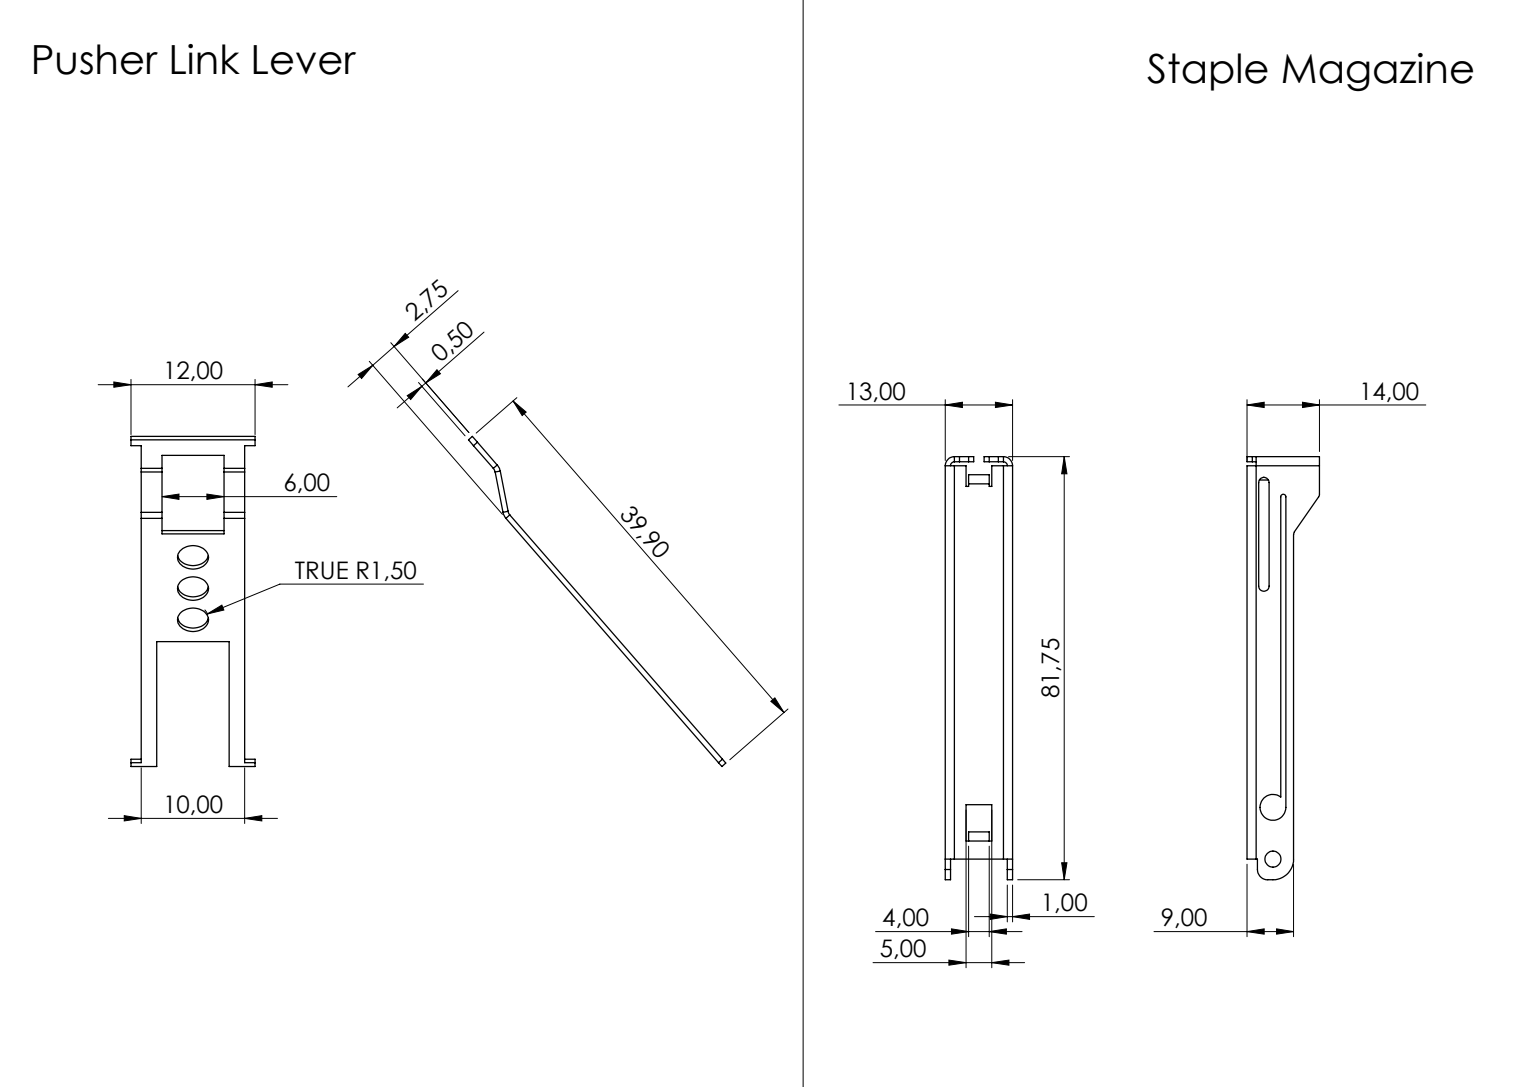
ISO-10303-21;
HEADER;
FILE_DESCRIPTION (('STEP AP214'),
    '1' );
FILE_NAME ('Staple Magazine.step',
    '2026-10-06T10:23:46',
    ( '' ),
    ( '' ),
    'SwSTEP 2.0',
    'SolidWorks 2020',
    '' );
FILE_SCHEMA (( 'AUTOMOTIVE_DESIGN' ));
ENDSEC;

DATA;
#2=ORIENTED_EDGE ( 'NONE', *, *, #5924, .T. ) ;
#11=DIRECTION ( 'NONE',  ( -6.056754644426120895E-31, -1.000000000000000000, -4.914813388431354887E-16 ) ) ;
#25=DIRECTION ( 'NONE',  ( 8.673617379884039170E-17, 2.999999999999999839E-15, 1.000000000000000000 ) ) ;
#29=EDGE_LOOP ( 'NONE', ( #453, #19107 ) ) ;
#33=CARTESIAN_POINT ( 'NONE',  ( 40.81606138205700773, -31.05876147765399864, 75.30501292737010033 ) ) ;
#40=CARTESIAN_POINT ( 'NONE',  ( 42.06606138205700063, 43.19123852234599781, 75.30501292736987295 ) ) ;
#46=( NAMED_UNIT ( * ) SI_UNIT ( $, .STERADIAN. ) SOLID_ANGLE_UNIT ( ) );
#53=ORIENTED_EDGE ( 'NONE', *, *, #21241, .F. ) ;
#64=VERTEX_POINT ( 'NONE', #911 ) ;
#66=EDGE_CURVE ( 'NONE', #3119, #2388, #6890, .T. ) ;
#78=FACE_BOUND ( 'NONE', #23310, .T. ) ;
#90=ORIENTED_EDGE ( 'NONE', *, *, #479, .T. ) ;
#93=AXIS2_PLACEMENT_3D ( 'NONE', #14032, #16324, #20207 ) ;
#94=EDGE_CURVE ( 'NONE', #4444, #1424, #20510, .T. ) ;
#95=DIRECTION ( 'NONE',  ( 1.000000000000000000, 0.000000000000000000, 0.000000000000000000 ) ) ;
#103=DIRECTION ( 'NONE',  ( 2.312964634635740294E-15, 2.999999999999999839E-15, 1.000000000000000000 ) ) ;
#108=VECTOR ( 'NONE', #19668, 1000.000000000000000 ) ;
#116=CARTESIAN_POINT ( 'NONE',  ( 44.81606138205700063, -24.55876147765401285, 70.30501292737008612 ) ) ;
#118=CYLINDRICAL_SURFACE ( 'NONE', #9476, 1.000000000000000888 ) ;
#132=AXIS2_PLACEMENT_3D ( 'NONE', #6490, #16519, #18844 ) ;
#141=EDGE_CURVE ( 'NONE', #14226, #13391, #3231, .T. ) ;
#150=AXIS2_PLACEMENT_3D ( 'NONE', #11257, #7991, #1314 ) ;
#154=VERTEX_POINT ( 'NONE', #12549 ) ;
#157=CARTESIAN_POINT ( 'NONE',  ( 36.31606138205700063, 39.69123852234597649, 69.30501292736988717 ) ) ;
#164=CIRCLE ( 'NONE', #21962, 1.000000000000000888 ) ;
#177=ORIENTED_EDGE ( 'NONE', *, *, #13046, .F. ) ;
#179=DIRECTION ( 'NONE',  ( 1.000000000000000000, -5.204170427930413997E-31, -1.734723475976804876E-16 ) ) ;
#186=ORIENTED_EDGE ( 'NONE', *, *, #12634, .T. ) ;
#197=VECTOR ( 'NONE', #7883, 1000.000000000000000 ) ;
#201=CARTESIAN_POINT ( 'NONE',  ( 44.81606138205700063, 41.44123852234595518, 61.30501292736988006 ) ) ;
#207=CARTESIAN_POINT ( 'NONE',  ( 40.31606138205700773, 37.94123852234599070, 73.55501292736988717 ) ) ;
#210=LINE ( 'NONE', #8213, #17640 ) ;
#216=EDGE_LOOP ( 'NONE', ( #18034, #25103, #6817, #21837 ) ) ;
#221=ORIENTED_EDGE ( 'NONE', *, *, #10919, .F. ) ;
#222=DIRECTION ( 'NONE',  ( 0.000000000000000000, -2.999999999999999839E-15, -1.000000000000000000 ) ) ;
#244=LINE ( 'NONE', #4267, #5670 ) ;
#245=EDGE_CURVE ( 'NONE', #15791, #17958, #9316, .T. ) ;
#254=CYLINDRICAL_SURFACE ( 'NONE', #13248, 1.000000000000000888 ) ;
#268=DIRECTION ( 'NONE',  ( 1.000000000000000000, 3.083952846180988900E-15, -3.854941057726327830E-16 ) ) ;
#270=CIRCLE ( 'NONE', #24538, 2.000000000000001776 ) ;
#278=ORIENTED_EDGE ( 'NONE', *, *, #24831, .T. ) ;
#285=CARTESIAN_POINT ( 'NONE',  ( 44.81606138205700063, -34.55876147765400930, 73.30501292737011454 ) ) ;
#293=CARTESIAN_POINT ( 'NONE',  ( 40.31606138205700773, 39.69123852234597649, 69.30501292736988717 ) ) ;
#294=DIRECTION ( 'NONE',  ( 0.000000000000000000, 2.775557561562888984E-15, 1.000000000000000000 ) ) ;
#297=DIRECTION ( 'NONE',  ( 0.000000000000000000, -2.999999999999999839E-15, -1.000000000000000000 ) ) ;
#302=FACE_OUTER_BOUND ( 'NONE', #11083, .T. ) ;
#304=ADVANCED_FACE ( 'NONE', ( #3366 ), #21151, .F. ) ;
#314=ORIENTED_EDGE ( 'NONE', *, *, #23269, .F. ) ;
#316=CARTESIAN_POINT ( 'NONE',  ( 40.31606138205700773, 38.69123852234599070, 73.55501292736988717 ) ) ;
#317=CARTESIAN_POINT ( 'NONE',  ( 31.81606138205700418, -24.55876147765401285, 70.30501292737008612 ) ) ;
#324=ORIENTED_EDGE ( 'NONE', *, *, #10135, .F. ) ;
#325=ORIENTED_EDGE ( 'NONE', *, *, #16629, .F. ) ;
#328=CARTESIAN_POINT ( 'NONE',  ( 31.81606138205700418, 28.69846577177642288, 66.12638289304319983 ) ) ;
#335=PLANE ( 'NONE',  #18029 ) ;
#342=ORIENTED_EDGE ( 'NONE', *, *, #16102, .F. ) ;
#347=DIRECTION ( 'NONE',  ( -3.717264591378870232E-16, -3.325260651745651169E-15, -1.000000000000000000 ) ) ;
#355=CARTESIAN_POINT ( 'NONE',  ( 33.56606138205700773, 41.44123852234599070, 73.55501292736987295 ) ) ;
#357=FACE_OUTER_BOUND ( 'NONE', #24183, .T. ) ;
#359=VECTOR ( 'NONE', #22680, 1000.000000000000000 ) ;
#363=EDGE_LOOP ( 'NONE', ( #20532, #24029, #12910, #14891, #19447, #20167, #13360, #10230, #14079, #1336, #8917 ) ) ;
#364=ORIENTED_EDGE ( 'NONE', *, *, #2300, .T. ) ;
#375=ADVANCED_FACE ( 'NONE', ( #8387 ), #5942, .F. ) ;
#384=CARTESIAN_POINT ( 'NONE',  ( 40.31606138205700773, 41.44123852234599781, 74.30501292736987295 ) ) ;
#392=CARTESIAN_POINT ( 'NONE',  ( 44.81606138205700063, -38.55876147765400930, 73.30501292737012875 ) ) ;
#409=EDGE_CURVE ( 'NONE', #17565, #5522, #244, .T. ) ;
#412=LINE ( 'NONE', #17964, #14177 ) ;
#428=ADVANCED_FACE ( 'NONE', ( #6197 ), #2308, .T. ) ;
#431=CARTESIAN_POINT ( 'NONE',  ( 36.31606138205700063, -30.30876147765400574, 73.55501292737010033 ) ) ;
#443=LINE ( 'NONE', #18607, #21420 ) ;
#444=LINE ( 'NONE', #22224, #5450 ) ;
#449=CARTESIAN_POINT ( 'NONE',  ( 35.31606138205687273, 42.19123852234595518, 61.80501292736988006 ) ) ;
#453=ORIENTED_EDGE ( 'NONE', *, *, #20893, .T. ) ;
#456=CARTESIAN_POINT ( 'NONE',  ( 36.31606138205700063, 43.19123852234599781, 74.30501292736987295 ) ) ;
#466=CARTESIAN_POINT ( 'NONE',  ( 33.56606138205700773, 43.19123852234599781, 75.30501292736987295 ) ) ;
#472=AXIS2_PLACEMENT_3D ( 'NONE', #1050, #9195, #18717 ) ;
#473=CARTESIAN_POINT ( 'NONE',  ( 31.81606138205700418, -22.55876147765401996, 68.80501292737008612 ) ) ;
#478=FACE_OUTER_BOUND ( 'NONE', #5733, .T. ) ;
#479=EDGE_CURVE ( 'NONE', #15938, #12825, #16471, .T. ) ;
#504=VECTOR ( 'NONE', #8993, 1000.000000000000000 ) ;
#515=CARTESIAN_POINT ( 'NONE',  ( 32.81606138205700773, 35.38401127291550097, 61.48364296169660292 ) ) ;
#518=AXIS2_PLACEMENT_3D ( 'NONE', #8054, #21699, #12437 ) ;
#531=FACE_OUTER_BOUND ( 'NONE', #15557, .T. ) ;
#537=FACE_OUTER_BOUND ( 'NONE', #20506, .T. ) ;
#540=CIRCLE ( 'NONE', #15353, 0.9999999999999940048 ) ;
#541=CARTESIAN_POINT ( 'NONE',  ( 31.81606138205700418, 38.19123852234599070, 72.05501292736988717 ) ) ;
#549=VECTOR ( 'NONE', #9794, 1000.000000000000000 ) ;
#555=AXIS2_PLACEMENT_3D ( 'NONE', #19698, #6310, #13908 ) ;
#570=DIRECTION ( 'NONE',  ( 0.000000000000000000, 1.000000000000000000, -2.999999999999999839E-15 ) ) ;
#595=DIRECTION ( 'NONE',  ( -1.836970198721029688E-16, -2.999999999999999839E-15, -1.000000000000000000 ) ) ;
#596=DIRECTION ( 'NONE',  ( 1.000000000000000000, -5.204170427930415223E-30, -1.734723475976805122E-15 ) ) ;
#620=ORIENTED_EDGE ( 'NONE', *, *, #4318, .T. ) ;
#646=ADVANCED_FACE ( 'NONE', ( #14389 ), #335, .T. ) ;
#652=EDGE_LOOP ( 'NONE', ( #17580, #11877, #24697, #22252 ) ) ;
#663=DIRECTION ( 'NONE',  ( 1.000000000000000000, 0.000000000000000000, 0.000000000000000000 ) ) ;
#665=LINE ( 'NONE', #21852, #15394 ) ;
#667=FACE_OUTER_BOUND ( 'NONE', #25437, .T. ) ;
#673=CARTESIAN_POINT ( 'NONE',  ( 34.56606138205700773, 41.44123852234599781, 74.30501292736987295 ) ) ;
#675=CARTESIAN_POINT ( 'NONE',  ( 36.31606138205700063, 37.44123852234599781, 74.30501292736988717 ) ) ;
#685=UNCERTAINTY_MEASURE_WITH_UNIT (LENGTH_MEASURE( 1.000000000000000082E-05 ), #25478, 'distance_accuracy_value', 'NONE');
#701=ORIENTED_EDGE ( 'NONE', *, *, #6875, .T. ) ;
#707=DIRECTION ( 'NONE',  ( -9.027796614315171564E-31, -1.000000000000000000, -3.938893903907230117E-15 ) ) ;
#712=VECTOR ( 'NONE', #15259, 1000.000000000000000 ) ;
#716=ORIENTED_EDGE ( 'NONE', *, *, #3484, .F. ) ;
#717=EDGE_CURVE ( 'NONE', #11800, #9537, #10630, .T. ) ;
#719=DIRECTION ( 'NONE',  ( 1.000000000000000000, 0.000000000000000000, 0.000000000000000000 ) ) ;
#737=DIRECTION ( 'NONE',  ( 3.469446951953614978E-15, 2.999999999999999839E-15, 1.000000000000000000 ) ) ;
#738=CARTESIAN_POINT ( 'NONE',  ( 44.81606138205700063, 18.19123852234599426, 73.05501292736995822 ) ) ;
#741=CARTESIAN_POINT ( 'NONE',  ( 31.81606138205700418, 38.19123852234599070, 73.05501292736988717 ) ) ;
#744=LINE ( 'NONE', #10175, #2475 ) ;
#745=ORIENTED_EDGE ( 'NONE', *, *, #978, .F. ) ;
#763=FACE_OUTER_BOUND ( 'NONE', #937, .T. ) ;
#767=ADVANCED_FACE ( 'NONE', ( #6412 ), #16191, .F. ) ;
#795=FACE_OUTER_BOUND ( 'NONE', #17917, .T. ) ;
#796=EDGE_CURVE ( 'NONE', #6775, #12825, #1233, .T. ) ;
#811=VECTOR ( 'NONE', #1544, 1000.000000000000000 ) ;
#821=VERTEX_POINT ( 'NONE', #16699 ) ;
#824=DIRECTION ( 'NONE',  ( 0.000000000000000000, -1.000000000000000000, 2.999999999999999839E-15 ) ) ;
#826=CARTESIAN_POINT ( 'NONE',  ( 31.81606138205700418, -34.55876147765401640, 70.30501292737011454 ) ) ;
#837=DIRECTION ( 'NONE',  ( -1.000000000000000000, 1.115179377413661005E-30, 3.717264591378870232E-16 ) ) ;
#842=ORIENTED_EDGE ( 'NONE', *, *, #1376, .F. ) ;
#875=DIRECTION ( 'NONE',  ( 3.491481338843135327E-15, 1.000000000000000000, -3.000000000000000628E-15 ) ) ;
#879=ORIENTED_EDGE ( 'NONE', *, *, #18939, .T. ) ;
#880=CIRCLE ( 'NONE', #9142, 1.000000000000000888 ) ;
#881=EDGE_CURVE ( 'NONE', #23679, #25358, #20565, .T. ) ;
#911=CARTESIAN_POINT ( 'NONE',  ( 43.81606138205700063, -24.55876147765401996, 67.80501292737008612 ) ) ;
#916=CARTESIAN_POINT ( 'NONE',  ( 32.81606138205700773, 38.19123852234599070, 72.05501292736988717 ) ) ;
#932=LINE ( 'NONE', #675, #6543 ) ;
#936=DIRECTION ( 'NONE',  ( 1.734723475976805122E-15, 2.999999999999999839E-15, 1.000000000000000000 ) ) ;
#937=EDGE_LOOP ( 'NONE', ( #6127, #19955, #5649, #11614 ) ) ;
#944=CARTESIAN_POINT ( 'NONE',  ( 36.31606138205700063, -31.05876147765400574, 73.55501292737010033 ) ) ;
#948=ORIENTED_EDGE ( 'NONE', *, *, #22550, .T. ) ;
#949=DIRECTION ( 'NONE',  ( -1.000000000000000000, 0.000000000000000000, 0.000000000000000000 ) ) ;
#950=VECTOR ( 'NONE', #22281, 1000.000000000000000 ) ;
#958=ORIENTED_EDGE ( 'NONE', *, *, #16247, .F. ) ;
#966=CARTESIAN_POINT ( 'NONE',  ( 43.06606138205700063, 41.44123852234595518, 61.30501292736988006 ) ) ;
#968=CARTESIAN_POINT ( 'NONE',  ( 31.81606138205700418, 18.19123852234598715, 71.05501292736995822 ) ) ;
#978=EDGE_CURVE ( 'NONE', #13410, #10587, #1600, .T. ) ;
#982=ORIENTED_EDGE ( 'NONE', *, *, #6042, .T. ) ;
#986=VECTOR ( 'NONE', #18996, 1000.000000000000000 ) ;
#987=CIRCLE ( 'NONE', #1749, 1.000000000000000888 ) ;
#1003=DIRECTION ( 'NONE',  ( 0.000000000000000000, 1.000000000000000000, 0.000000000000000000 ) ) ;
#1006=AXIS2_PLACEMENT_3D ( 'NONE', #18778, #9324, #5440 ) ;
#1010=CARTESIAN_POINT ( 'NONE',  ( 40.31606138205700773, 37.94123852234599781, 74.30501292736988717 ) ) ;
#1016=VECTOR ( 'NONE', #24571, 1000.000000000000000 ) ;
#1019=DIRECTION ( 'NONE',  ( -1.000000000000000000, 0.000000000000000000, 0.000000000000000000 ) ) ;
#1022=EDGE_CURVE ( 'NONE', #11745, #2525, #15272, .T. ) ;
#1033=CARTESIAN_POINT ( 'NONE',  ( 38.31606138205700063, -30.30876147765400574, 72.30501292737010033 ) ) ;
#1036=EDGE_LOOP ( 'NONE', ( #23616, #23189, #2368, #21937 ) ) ;
#1050=CARTESIAN_POINT ( 'NONE',  ( 44.81606138205700063, -24.55876147765401285, 70.30501292737008612 ) ) ;
#1055=ORIENTED_EDGE ( 'NONE', *, *, #5647, .F. ) ;
#1066=ORIENTED_EDGE ( 'NONE', *, *, #22005, .T. ) ;
#1074=EDGE_LOOP ( 'NONE', ( #6439, #18112, #14922, #14485 ) ) ;
#1084=ORIENTED_EDGE ( 'NONE', *, *, #10520, .F. ) ;
#1086=DIRECTION ( 'NONE',  ( -1.000000000000000000, 5.510910596163088391E-31, 1.836970198721029688E-16 ) ) ;
#1094=CARTESIAN_POINT ( 'NONE',  ( 31.81606138205700418, -34.55876147765401640, 70.30501292737011454 ) ) ;
#1107=DIRECTION ( 'NONE',  ( -1.000000000000000000, 5.204170427930415223E-30, 1.734723475976805122E-15 ) ) ;
#1119=EDGE_CURVE ( 'NONE', #5642, #11800, #12204, .T. ) ;
#1129=ORIENTED_EDGE ( 'NONE', *, *, #18715, .T. ) ;
#1142=VERTEX_POINT ( 'NONE', #22358 ) ;
#1155=CARTESIAN_POINT ( 'NONE',  ( 31.81606138205700418, -34.55876147765401640, 70.30501292737011454 ) ) ;
#1173=VECTOR ( 'NONE', #6959, 1000.000000000000000 ) ;
#1175=AXIS2_PLACEMENT_3D ( 'NONE', #24620, #8563, #4942 ) ;
#1180=EDGE_CURVE ( 'NONE', #7272, #21608, #20308, .T. ) ;
#1183=DIRECTION ( 'NONE',  ( 0.000000000000000000, 0.5703958094953464064, 0.8213699656732943444 ) ) ;
#1187=DIRECTION ( 'NONE',  ( 0.000000000000000000, -1.000000000000000000, 2.999999999999999839E-15 ) ) ;
#1192=COLOUR_RGB ( '', 0.31764706, 0.68627451, 0.89019608) ;
#1195=AXIS2_PLACEMENT_3D ( 'NONE', #20880, #3219, #19198 ) ;
#1196=EDGE_CURVE ( 'NONE', #13325, #17789, #3167, .T. ) ;
#1198=ORIENTED_EDGE ( 'NONE', *, *, #14465, .F. ) ;
#1199=VERTEX_POINT ( 'NONE', #12332 ) ;
#1210=VECTOR ( 'NONE', #15431, 1000.000000000000000 ) ;
#1214=ORIENTED_EDGE ( 'NONE', *, *, #12103, .F. ) ;
#1215=EDGE_CURVE ( 'NONE', #21718, #13011, #24273, .T. ) ;
#1225=AXIS2_PLACEMENT_3D ( 'NONE', #6385, #8318, #16034 ) ;
#1227=ORIENTED_EDGE ( 'NONE', *, *, #6032, .F. ) ;
#1230=LINE ( 'NONE', #8371, #20694 ) ;
#1231=AXIS2_PLACEMENT_3D ( 'NONE', #23636, #18106, #21584 ) ;
#1233=LINE ( 'NONE', #1359, #7332 ) ;
#1236=FACE_OUTER_BOUND ( 'NONE', #11990, .T. ) ;
#1244=VERTEX_POINT ( 'NONE', #17079 ) ;
#1246=LINE ( 'NONE', #9127, #504 ) ;
#1259=DIRECTION ( 'NONE',  ( 0.000000000000000000, 1.000000000000000000, -5.551115123125785858E-15 ) ) ;
#1263=ORIENTED_EDGE ( 'NONE', *, *, #4909, .F. ) ;
#1264=VECTOR ( 'NONE', #4201, 1000.000000000000000 ) ;
#1268=ORIENTED_EDGE ( 'NONE', *, *, #6443, .F. ) ;
#1281=FACE_OUTER_BOUND ( 'NONE', #17840, .T. ) ;
#1290=ORIENTED_EDGE ( 'NONE', *, *, #23271, .T. ) ;
#1298=ORIENTED_EDGE ( 'NONE', *, *, #21210, .T. ) ;
#1314=DIRECTION ( 'NONE',  ( 1.189524669241238159E-14, 1.000000000000000000, -3.965082230804126670E-15 ) ) ;
#1319=SHAPE_DEFINITION_REPRESENTATION ( #23060, #7525 ) ;
#1333=DIRECTION ( 'NONE',  ( -1.000000000000000000, 5.204170427930415223E-30, 1.734723475976805122E-15 ) ) ;
#1336=ORIENTED_EDGE ( 'NONE', *, *, #19490, .T. ) ;
#1350=VECTOR ( 'NONE', #7285, 1000.000000000000000 ) ;
#1352=DIRECTION ( 'NONE',  ( -1.000000000000000000, 1.115179377413661005E-30, 3.717264591378870232E-16 ) ) ;
#1359=CARTESIAN_POINT ( 'NONE',  ( 38.31606138205700063, -29.30876147765400574, 73.55501292737010033 ) ) ;
#1362=FACE_OUTER_BOUND ( 'NONE', #24504, .T. ) ;
#1363=VERTEX_POINT ( 'NONE', #4965 ) ;
#1367=ADVANCED_FACE ( 'NONE', ( #22480 ), #8716, .F. ) ;
#1376=EDGE_CURVE ( 'NONE', #15787, #6943, #9101, .T. ) ;
#1379=DIRECTION ( 'NONE',  ( 1.000000000000000000, 1.289685230616452080E-30, -8.343550184191211817E-45 ) ) ;
#1381=VECTOR ( 'NONE', #22924, 1000.000000000000000 ) ;
#1389=CARTESIAN_POINT ( 'NONE',  ( 44.81606138205700063, -24.55876147765401285, 70.30501292737008612 ) ) ;
#1390=CIRCLE ( 'NONE', #150, 1.750000000000001554 ) ;
#1394=CARTESIAN_POINT ( 'NONE',  ( 41.31606138205687273, 42.19123852234595518, 61.80501292736988006 ) ) ;
#1397=EDGE_LOOP ( 'NONE', ( #14568, #17357, #12669, #9728 ) ) ;
#1398=ORIENTED_EDGE ( 'NONE', *, *, #6590, .T. ) ;
#1405=CARTESIAN_POINT ( 'NONE',  ( 33.56606138205700773, 41.44123852234599070, 73.55501292736987295 ) ) ;
#1406=CARTESIAN_POINT ( 'NONE',  ( 43.81606138205700063, 35.95440708241085304, 61.30501292736990138 ) ) ;
#1413=ADVANCED_FACE ( 'NONE', ( #13587 ), #23234, .T. ) ;
#1415=AXIS2_PLACEMENT_3D ( 'NONE', #23739, #15501, #6104 ) ;
#1419=ORIENTED_EDGE ( 'NONE', *, *, #5165, .F. ) ;
#1420=CARTESIAN_POINT ( 'NONE',  ( 38.31606138205700063, 39.69123852234599070, 73.55501292736988717 ) ) ;
#1424=VERTEX_POINT ( 'NONE', #15383 ) ;
#1429=ORIENTED_EDGE ( 'NONE', *, *, #14272, .T. ) ;
#1434=EDGE_LOOP ( 'NONE', ( #2248, #19526, #19970, #6158 ) ) ;
#1441=DIRECTION ( 'NONE',  ( 3.717264591378870232E-16, 2.999999999999999839E-15, 1.000000000000000000 ) ) ;
#1444=ORIENTED_EDGE ( 'NONE', *, *, #20014, .F. ) ;
#1452=CARTESIAN_POINT ( 'NONE',  ( 33.56606138205700773, 43.19123852234599070, 73.55501292736987295 ) ) ;
#1457=ORIENTED_EDGE ( 'NONE', *, *, #2541, .T. ) ;
#1461=LINE ( 'NONE', #5711, #20288 ) ;
#1465=DIRECTION ( 'NONE',  ( 1.000000000000000000, 0.000000000000000000, 0.000000000000000000 ) ) ;
#1473=ORIENTED_EDGE ( 'NONE', *, *, #15238, .T. ) ;
#1483=CARTESIAN_POINT ( 'NONE',  ( 33.56606138205700773, 41.44123852234595518, 61.30501292736988006 ) ) ;
#1484=ORIENTED_EDGE ( 'NONE', *, *, #21527, .F. ) ;
#1503=CARTESIAN_POINT ( 'NONE',  ( 37.31606138205700063, 43.19123852234599070, 73.55501292736987295 ) ) ;
#1511=ORIENTED_EDGE ( 'NONE', *, *, #22943, .F. ) ;
#1513=EDGE_CURVE ( 'NONE', #4468, #8243, #13715, .T. ) ;
#1521=FACE_BOUND ( 'NONE', #18539, .T. ) ;
#1528=EDGE_CURVE ( 'NONE', #14570, #22793, #25149, .T. ) ;
#1531=EDGE_CURVE ( 'NONE', #4589, #5235, #15503, .T. ) ;
#1540=EDGE_CURVE ( 'NONE', #13029, #21703, #21191, .T. ) ;
#1544=DIRECTION ( 'NONE',  ( 3.540251991789399939E-16, 2.999999999999999839E-15, 1.000000000000000000 ) ) ;
#1558=ORIENTED_EDGE ( 'NONE', *, *, #20114, .F. ) ;
#1572=CARTESIAN_POINT ( 'NONE',  ( 31.81606138205700418, 35.95440708241085304, 61.30501292736990138 ) ) ;
#1576=ORIENTED_EDGE ( 'NONE', *, *, #7200, .F. ) ;
#1582=EDGE_CURVE ( 'NONE', #24731, #3483, #24567, .T. ) ;
#1584=ADVANCED_FACE ( 'NONE', ( #667 ), #6368, .F. ) ;
#1589=ORIENTED_EDGE ( 'NONE', *, *, #16586, .F. ) ;
#1590=DIRECTION ( 'NONE',  ( 0.000000000000000000, -1.000000000000000000, 2.999999999999999839E-15 ) ) ;
#1592=ORIENTED_EDGE ( 'NONE', *, *, #18681, .F. ) ;
#1600=LINE ( 'NONE', #17593, #4409 ) ;
#1623=DIRECTION ( 'NONE',  ( 0.000000000000000000, -1.000000000000000000, 0.000000000000000000 ) ) ;
#1624=VECTOR ( 'NONE', #6871, 1000.000000000000000 ) ;
#1635=AXIS2_PLACEMENT_3D ( 'NONE', #25363, #15341, #3873 ) ;
#1636=PLANE ( 'NONE',  #3783 ) ;
#1645=CARTESIAN_POINT ( 'NONE',  ( 38.31606138205700063, 39.69123852234599781, 75.30501292737004349 ) ) ;
#1649=LINE ( 'NONE', #19193, #18066 ) ;
#1652=AXIS2_PLACEMENT_3D ( 'NONE', #11685, #11808, #15407 ) ;
#1656=LINE ( 'NONE', #5419, #7800 ) ;
#1665=CARTESIAN_POINT ( 'NONE',  ( 36.31606138205700063, 42.19123852234599781, 74.30501292736987295 ) ) ;
#1671=LINE ( 'NONE', #25110, #14190 ) ;
#1672=LINE ( 'NONE', #11757, #23163 ) ;
#1681=ORIENTED_EDGE ( 'NONE', *, *, #10661, .T. ) ;
#1689=CYLINDRICAL_SURFACE ( 'NONE', #24607, 1.750000000000001554 ) ;
#1692=EDGE_CURVE ( 'NONE', #4589, #20194, #18093, .T. ) ;
#1698=CARTESIAN_POINT ( 'NONE',  ( 43.06606138205700063, 43.19123852234599781, 74.30501292736987295 ) ) ;
#1699=DIRECTION ( 'NONE',  ( 1.000000000000000000, 0.000000000000000000, 0.000000000000000000 ) ) ;
#1708=CARTESIAN_POINT ( 'NONE',  ( 43.06606138205700063, 43.19123852234599070, 73.55501292736987295 ) ) ;
#1712=ORIENTED_EDGE ( 'NONE', *, *, #6965, .F. ) ;
#1714=DIRECTION ( 'NONE',  ( 0.000000000000000000, -2.999999999999999839E-15, -1.000000000000000000 ) ) ;
#1727=VERTEX_POINT ( 'NONE', #20013 ) ;
#1740=CYLINDRICAL_SURFACE ( 'NONE', #8286, 3.999999999999996447 ) ;
#1742=FACE_OUTER_BOUND ( 'NONE', #23140, .T. ) ;
#1744=VECTOR ( 'NONE', #6544, 1000.000000000000000 ) ;
#1749=AXIS2_PLACEMENT_3D ( 'NONE', #22322, #6608, #14002 ) ;
#1751=CIRCLE ( 'NONE', #15334, 1.000000000000000888 ) ;
#1761=EDGE_CURVE ( 'NONE', #19667, #17699, #12931, .T. ) ;
#1763=ORIENTED_EDGE ( 'NONE', *, *, #12811, .F. ) ;
#1773=FACE_OUTER_BOUND ( 'NONE', #6985, .T. ) ;
#1774=DIRECTION ( 'NONE',  ( -0.000000000000000000, -1.000000000000000000, 2.848211695852029218E-15 ) ) ;
#1776=AXIS2_PLACEMENT_3D ( 'NONE', #23319, #11499, #23452 ) ;
#1779=FACE_OUTER_BOUND ( 'NONE', #18015, .T. ) ;
#1781=DIRECTION ( 'NONE',  ( 0.000000000000000000, -2.999999999999999839E-15, -1.000000000000000000 ) ) ;
#1782=AXIS2_PLACEMENT_3D ( 'NONE', #13346, #1714, #17204 ) ;
#1789=ORIENTED_EDGE ( 'NONE', *, *, #10064, .F. ) ;
#1791=VECTOR ( 'NONE', #10771, 1000.000000000000000 ) ;
#1803=PLANE ( 'NONE',  #18725 ) ;
#1804=PLANE ( 'NONE',  #19891 ) ;
#1813=VECTOR ( 'NONE', #15382, 1000.000000000000000 ) ;
#1823=EDGE_CURVE ( 'NONE', #20324, #10597, #10869, .T. ) ;
#1826=EDGE_CURVE ( 'NONE', #13483, #15432, #7333, .T. ) ;
#1831=ORIENTED_EDGE ( 'NONE', *, *, #1531, .F. ) ;
#1840=EDGE_CURVE ( 'NONE', #8848, #12037, #13918, .T. ) ;
#1857=ADVANCED_FACE ( 'NONE', ( #795 ), #12802, .F. ) ;
#1864=DIRECTION ( 'NONE',  ( 1.000000000000000000, 0.000000000000000000, 0.000000000000000000 ) ) ;
#1872=ADVANCED_FACE ( 'NONE', ( #22701 ), #10741, .T. ) ;
#1873=CARTESIAN_POINT ( 'NONE',  ( 43.06606138205700063, -34.55876147765401640, 70.30501292737011454 ) ) ;
#1877=VERTEX_POINT ( 'NONE', #20646 ) ;
#1887=CARTESIAN_POINT ( 'NONE',  ( 44.81606138205700063, 41.44123852234595518, 61.30501292736988006 ) ) ;
#1889=CARTESIAN_POINT ( 'NONE',  ( 33.56606138205700773, -34.55876147765400930, 73.55501292737011454 ) ) ;
#1894=DIRECTION ( 'NONE',  ( -1.000000000000000000, 0.000000000000000000, 0.000000000000000000 ) ) ;
#1902=SURFACE_SIDE_STYLE ('',( #23682 ) ) ;
#1907=ORIENTED_EDGE ( 'NONE', *, *, #13379, .F. ) ;
#1926=VECTOR ( 'NONE', #21980, 1000.000000000000000 ) ;
#1931=ORIENTED_EDGE ( 'NONE', *, *, #5771, .T. ) ;
#1940=LINE ( 'NONE', #5826, #14696 ) ;
#1945=CIRCLE ( 'NONE', #24957, 1.750000000000001554 ) ;
#1952=ORIENTED_EDGE ( 'NONE', *, *, #16632, .F. ) ;
#1954=VERTEX_POINT ( 'NONE', #22833 ) ;
#1960=CYLINDRICAL_SURFACE ( 'NONE', #21172, 1.000000000000000888 ) ;
#1966=AXIS2_PLACEMENT_3D ( 'NONE', #12340, #8340, #17621 ) ;
#1969=CARTESIAN_POINT ( 'NONE',  ( 33.56606138205700773, 41.44123852234599070, 73.55501292736987295 ) ) ;
#1975=( NAMED_UNIT ( * ) PLANE_ANGLE_UNIT ( ) SI_UNIT ( $, .RADIAN. ) );
#1987=ORIENTED_EDGE ( 'NONE', *, *, #23271, .F. ) ;
#1988=DIRECTION ( 'NONE',  ( -8.673617379884039170E-17, 1.163336342344335610E-15, -1.000000000000000000 ) ) ;
#2000=AXIS2_PLACEMENT_3D ( 'NONE', #9286, #12766, #22537 ) ;
#2010=ORIENTED_EDGE ( 'NONE', *, *, #4137, .F. ) ;
#2011=VECTOR ( 'NONE', #5994, 1000.000000000000000 ) ;
#2016=AXIS2_PLACEMENT_3D ( 'NONE', #11059, #22397, #20344 ) ;
#2023=ORIENTED_EDGE ( 'NONE', *, *, #19159, .F. ) ;
#2030=CARTESIAN_POINT ( 'NONE',  ( 33.56606138205700773, 42.19123852234599070, 73.55501292736987295 ) ) ;
#2037=VECTOR ( 'NONE', #2768, 1000.000000000000000 ) ;
#2043=VECTOR ( 'NONE', #9012, 1000.000000000000000 ) ;
#2093=DIRECTION ( 'NONE',  ( 0.000000000000000000, 2.999999999999999839E-15, 1.000000000000000000 ) ) ;
#2098=EDGE_CURVE ( 'NONE', #5909, #19241, #12645, .T. ) ;
#2113=LINE ( 'NONE', #24002, #23315 ) ;
#2115=DIRECTION ( 'NONE',  ( 1.209079903702923825E-31, -1.000000000000000000, 3.325260651745651169E-15 ) ) ;
#2125=EDGE_LOOP ( 'NONE', ( #16708, #15029, #1457, #1398 ) ) ;
#2128=VECTOR ( 'NONE', #7850, 1000.000000000000000 ) ;
#2150=ORIENTED_EDGE ( 'NONE', *, *, #4100, .F. ) ;
#2158=FACE_OUTER_BOUND ( 'NONE', #8481, .T. ) ;
#2161=ORIENTED_EDGE ( 'NONE', *, *, #22066, .T. ) ;
#2171=LINE ( 'NONE', #15953, #13139 ) ;
#2180=EDGE_LOOP ( 'NONE', ( #1763, #24910, #20575, #23053 ) ) ;
#2181=ORIENTED_EDGE ( 'NONE', *, *, #18945, .F. ) ;
#2194=EDGE_CURVE ( 'NONE', #8063, #11585, #13719, .T. ) ;
#2197=DIRECTION ( 'NONE',  ( 0.000000000000000000, 2.999999999999999839E-15, 1.000000000000000000 ) ) ;
#2199=DIRECTION ( 'NONE',  ( -1.000000000000000000, 5.204170427930413997E-31, 1.734723475976804876E-16 ) ) ;
#2203=EDGE_CURVE ( 'NONE', #154, #2408, #9356, .T. ) ;
#2212=LINE ( 'NONE', #16120, #11823 ) ;
#2223=ORIENTED_EDGE ( 'NONE', *, *, #11008, .T. ) ;
#2228=PLANE ( 'NONE',  #24849 ) ;
#2236=CARTESIAN_POINT ( 'NONE',  ( 32.81606138205700773, -24.55876147765401285, 70.30501292737008612 ) ) ;
#2239=PLANE ( 'NONE',  #7123 ) ;
#2248=ORIENTED_EDGE ( 'NONE', *, *, #17169, .F. ) ;
#2258=ORIENTED_EDGE ( 'NONE', *, *, #6571, .F. ) ;
#2273=CARTESIAN_POINT ( 'NONE',  ( 36.31606138205700063, -31.05876147765400574, 73.55501292737010033 ) ) ;
#2300=EDGE_CURVE ( 'NONE', #1142, #13410, #11797, .T. ) ;
#2301=DIRECTION ( 'NONE',  ( -3.083952846180990083E-15, 1.000000000000000000, -2.999999999999998655E-15 ) ) ;
#2308=PLANE ( 'NONE',  #16359 ) ;
#2309=VERTEX_POINT ( 'NONE', #5602 ) ;
#2310=DIRECTION ( 'NONE',  ( 1.836970198721029688E-16, 2.999999999999999839E-15, 1.000000000000000000 ) ) ;
#2318=ADVANCED_FACE ( 'NONE', ( #13594 ), #21444, .T. ) ;
#2320=EDGE_CURVE ( 'NONE', #23734, #16934, #7796, .T. ) ;
#2329=LINE ( 'NONE', #392, #6554 ) ;
#2343=ORIENTED_EDGE ( 'NONE', *, *, #13920, .T. ) ;
#2359=DIRECTION ( 'NONE',  ( 1.000000000000000000, -3.083952846180990083E-15, 9.251858538542970050E-30 ) ) ;
#2365=ORIENTED_EDGE ( 'NONE', *, *, #10064, .T. ) ;
#2367=VERTEX_POINT ( 'NONE', #18099 ) ;
#2368=ORIENTED_EDGE ( 'NONE', *, *, #21667, .F. ) ;
#2371=DIRECTION ( 'NONE',  ( -9.027796614315171564E-31, -1.000000000000000000, -3.938893903907230117E-15 ) ) ;
#2383=CARTESIAN_POINT ( 'NONE',  ( 43.81606138205700063, -33.00876147765401925, 70.30501292737011454 ) ) ;
#2388=VERTEX_POINT ( 'NONE', #8301 ) ;
#2393=CARTESIAN_POINT ( 'NONE',  ( 40.31606138205700773, -31.05876147765399864, 75.30501292737008612 ) ) ;
#2394=DIRECTION ( 'NONE',  ( 1.000000000000000000, 0.000000000000000000, 0.000000000000000000 ) ) ;
#2407=EDGE_CURVE ( 'NONE', #12138, #13165, #17997, .T. ) ;
#2408=VERTEX_POINT ( 'NONE', #14228 ) ;
#2412=CIRCLE ( 'NONE', #16825, 1.000000000000000888 ) ;
#2416=DIRECTION ( 'NONE',  ( -9.027796614315171564E-31, -1.000000000000000000, -3.938893903907230117E-15 ) ) ;
#2418=ADVANCED_FACE ( 'NONE', ( #15891 ), #6372, .F. ) ;
#2419=CARTESIAN_POINT ( 'NONE',  ( 38.31606138205700063, -30.30876147765401996, 69.30501292737010033 ) ) ;
#2427=FACE_OUTER_BOUND ( 'NONE', #23941, .T. ) ;
#2428=CARTESIAN_POINT ( 'NONE',  ( 31.81606138205700418, -24.55876147765401996, 67.80501292737008612 ) ) ;
#2432=CIRCLE ( 'NONE', #5738, 2.000000000000001776 ) ;
#2434=DIRECTION ( 'NONE',  ( -1.000000000000000000, 1.301042606982604506E-30, 4.336808689942015271E-16 ) ) ;
#2438=ORIENTED_EDGE ( 'NONE', *, *, #9873, .T. ) ;
#2448=CIRCLE ( 'NONE', #20155, 1.750000000000001554 ) ;
#2462=ORIENTED_EDGE ( 'NONE', *, *, #10200, .T. ) ;
#2471=ORIENTED_EDGE ( 'NONE', *, *, #8526, .F. ) ;
#2472=FACE_OUTER_BOUND ( 'NONE', #17154, .T. ) ;
#2475=VECTOR ( 'NONE', #10305, 1000.000000000000000 ) ;
#2485=DIRECTION ( 'NONE',  ( -3.083952846180990083E-15, -1.000000000000000000, 2.999999999999999839E-15 ) ) ;
#2490=DIRECTION ( 'NONE',  ( 0.000000000000000000, 1.000000000000000000, -3.469446951953614189E-15 ) ) ;
#2492=LINE ( 'NONE', #16276, #13869 ) ;
#2509=DIRECTION ( 'NONE',  ( 1.514188661106530005E-31, 1.000000000000000000, -2.999999999999999839E-15 ) ) ;
#2516=LINE ( 'NONE', #10397, #8144 ) ;
#2524=LINE ( 'NONE', #466, #7852 ) ;
#2525=VERTEX_POINT ( 'NONE', #7126 ) ;
#2526=ORIENTED_EDGE ( 'NONE', *, *, #9282, .T. ) ;
#2540=AXIS2_PLACEMENT_3D ( 'NONE', #22311, #11074, #21118 ) ;
#2541=EDGE_CURVE ( 'NONE', #16347, #15938, #6745, .T. ) ;
#2560=DIRECTION ( 'NONE',  ( -1.000000000000000000, 1.115179377413661005E-30, 3.717264591378870232E-16 ) ) ;
#2561=AXIS2_PLACEMENT_3D ( 'NONE', #3982, #21505, #3856 ) ;
#2576=AXIS2_PLACEMENT_3D ( 'NONE', #3929, #9485, #9616 ) ;
#2588=ORIENTED_EDGE ( 'NONE', *, *, #25480, .T. ) ;
#2597=DIRECTION ( 'NONE',  ( 0.000000000000000000, -1.000000000000000000, 2.999999999999999839E-15 ) ) ;
#2628=LINE ( 'NONE', #2743, #6750 ) ;
#2632=EDGE_LOOP ( 'NONE', ( #5538, #17725, #314, #8172 ) ) ;
#2638=MECHANICAL_DESIGN_GEOMETRIC_PRESENTATION_REPRESENTATION('',(#21575),#8410);
#2641=VECTOR ( 'NONE', #11145, 1000.000000000000000 ) ;
#2661=EDGE_LOOP ( 'NONE', ( #20431, #5111, #22527, #13345 ) ) ;
#2662=ORIENTED_EDGE ( 'NONE', *, *, #14826, .F. ) ;
#2669=DIRECTION ( 'NONE',  ( 0.000000000000000000, -6.938893903907222067E-15, 1.000000000000000000 ) ) ;
#2672=AXIS2_PLACEMENT_3D ( 'NONE', #13302, #25245, #25371 ) ;
#2675=CARTESIAN_POINT ( 'NONE',  ( 38.31606138205700063, 42.51966564709218943, 72.30501292737018559 ) ) ;
#2676=ORIENTED_EDGE ( 'NONE', *, *, #22313, .T. ) ;
#2678=CARTESIAN_POINT ( 'NONE',  ( 32.81606138205700773, 38.19123852234598360, 71.05501292736988717 ) ) ;
#2680=ORIENTED_EDGE ( 'NONE', *, *, #4318, .F. ) ;
#2688=ORIENTED_EDGE ( 'NONE', *, *, #13968, .F. ) ;
#2689=CARTESIAN_POINT ( 'NONE',  ( 33.56606138205700773, -34.55876147765400219, 74.30501292737011454 ) ) ;
#2690=EDGE_CURVE ( 'NONE', #10464, #19274, #1940, .T. ) ;
#2699=EDGE_CURVE ( 'NONE', #14226, #16502, #9576, .T. ) ;
#2700=PLANE ( 'NONE',  #4278 ) ;
#2705=ORIENTED_EDGE ( 'NONE', *, *, #9826, .F. ) ;
#2707=DIRECTION ( 'NONE',  ( 0.000000000000000000, 1.000000000000000000, 0.000000000000000000 ) ) ;
#2717=PLANE ( 'NONE',  #19942 ) ;
#2720=FACE_OUTER_BOUND ( 'NONE', #3411, .T. ) ;
#2727=EDGE_CURVE ( 'NONE', #2309, #19667, #11509, .T. ) ;
#2733=VECTOR ( 'NONE', #12443, 1000.000000000000000 ) ;
#2743=CARTESIAN_POINT ( 'NONE',  ( 38.31606138205712853, 42.19123852234596939, 65.30501292736988717 ) ) ;
#2749=CARTESIAN_POINT ( 'NONE',  ( 43.06606138205700063, 41.44123852234599781, 74.30501292736987295 ) ) ;
#2768=DIRECTION ( 'NONE',  ( 0.000000000000000000, 1.000000000000000000, -3.325260651745651169E-15 ) ) ;
#2774=ORIENTED_EDGE ( 'NONE', *, *, #25480, .F. ) ;
#2778=EDGE_CURVE ( 'NONE', #21084, #9967, #9825, .T. ) ;
#2780=ORIENTED_EDGE ( 'NONE', *, *, #6442, .F. ) ;
#2781=ORIENTED_EDGE ( 'NONE', *, *, #13984, .F. ) ;
#2790=VECTOR ( 'NONE', #13100, 1000.000000000000000 ) ;
#2792=AXIS2_PLACEMENT_3D ( 'NONE', #3118, #14843, #14713 ) ;
#2794=DIRECTION ( 'NONE',  ( 1.000000000000000000, 0.000000000000000000, 0.000000000000000000 ) ) ;
#2802=CARTESIAN_POINT ( 'NONE',  ( 41.81606138205687273, 43.19123852234595518, 61.30501292736988006 ) ) ;
#2804=CARTESIAN_POINT ( 'NONE',  ( 34.81606138205687273, 42.19123852234595518, 61.80501292736988006 ) ) ;
#2806=VERTEX_POINT ( 'NONE', #14442 ) ;
#2809=VECTOR ( 'NONE', #9333, 1000.000000000000000 ) ;
#2815=CARTESIAN_POINT ( 'NONE',  ( 36.31606138205700063, -29.30876147765401640, 69.30501292737010033 ) ) ;
#2831=EDGE_LOOP ( 'NONE', ( #8003, #6092, #22375, #12048 ) ) ;
#2832=AXIS2_PLACEMENT_3D ( 'NONE', #1094, #16828, #24412 ) ;
#2840=FACE_OUTER_BOUND ( 'NONE', #24503, .T. ) ;
#2859=CARTESIAN_POINT ( 'NONE',  ( 39.31606138205700063, 43.19123852234599781, 75.30501292736987295 ) ) ;
#2875=ORIENTED_EDGE ( 'NONE', *, *, #94, .T. ) ;
#2884=DIRECTION ( 'NONE',  ( 1.000000000000000000, 0.000000000000000000, 0.000000000000000000 ) ) ;
#2885=ORIENTED_EDGE ( 'NONE', *, *, #2407, .F. ) ;
#2888=LINE ( 'NONE', #19379, #1350 ) ;
#2891=VERTEX_POINT ( 'NONE', #515 ) ;
#2893=PLANE ( 'NONE',  #19862 ) ;
#2895=ORIENTED_EDGE ( 'NONE', *, *, #22511, .F. ) ;
#2898=DIRECTION ( 'NONE',  ( 1.000000000000000000, 1.115287202090205222E-30, -1.734723475976805122E-15 ) ) ;
#2902=DIRECTION ( 'NONE',  ( 1.000000000000000000, 0.000000000000000000, 0.000000000000000000 ) ) ;
#2910=ORIENTED_EDGE ( 'NONE', *, *, #12103, .T. ) ;
#2925=EDGE_CURVE ( 'NONE', #19241, #4343, #13082, .T. ) ;
#2927=EDGE_CURVE ( 'NONE', #12825, #17958, #1945, .T. ) ;
#2935=ADVANCED_FACE ( 'NONE', ( #10199 ), #14315, .T. ) ;
#2954=DIRECTION ( 'NONE',  ( 0.000000000000000000, 1.000000000000000000, -2.999999999999998655E-15 ) ) ;
#2979=CARTESIAN_POINT ( 'NONE',  ( 40.31606138205700773, 38.69123852234599781, 75.30501292737004349 ) ) ;
#2992=CYLINDRICAL_SURFACE ( 'NONE', #14533, 1.000000000000000888 ) ;
#3000=EDGE_LOOP ( 'NONE', ( #2526, #7354, #10115, #4750 ) ) ;
#3003=DIRECTION ( 'NONE',  ( 0.000000000000000000, -6.938893903907222067E-15, 1.000000000000000000 ) ) ;
#3021=ORIENTED_EDGE ( 'NONE', *, *, #1196, .F. ) ;
#3027=CIRCLE ( 'NONE', #19491, 1.000000000000000888 ) ;
#3028=CARTESIAN_POINT ( 'NONE',  ( 36.31606138205700063, 37.94123852234599781, 74.30501292736988717 ) ) ;
#3048=CIRCLE ( 'NONE', #6776, 1.000000000000000888 ) ;
#3050=DIRECTION ( 'NONE',  ( 0.000000000000000000, 1.000000000000000000, -2.999999999999999839E-15 ) ) ;
#3053=FACE_OUTER_BOUND ( 'NONE', #17960, .T. ) ;
#3060=LINE ( 'NONE', #10936, #6085 ) ;
#3077=DIRECTION ( 'NONE',  ( -1.000000000000000000, -6.938893903907222067E-15, 0.000000000000000000 ) ) ;
#3080=VECTOR ( 'NONE', #19562, 1000.000000000000000 ) ;
#3094=ORIENTED_EDGE ( 'NONE', *, *, #9813, .F. ) ;
#3101=ORIENTED_EDGE ( 'NONE', *, *, #20873, .F. ) ;
#3112=EDGE_CURVE ( 'NONE', #17565, #20324, #12778, .T. ) ;
#3118=CARTESIAN_POINT ( 'NONE',  ( 36.31606138205700063, 37.94123852234599070, 73.55501292736988717 ) ) ;
#3119=VERTEX_POINT ( 'NONE', #7223 ) ;
#3128=CARTESIAN_POINT ( 'NONE',  ( 31.81606138205700418, 41.44123852234595518, 61.30501292736988006 ) ) ;
#3130=LINE ( 'NONE', #4575, #2733 ) ;
#3140=VERTEX_POINT ( 'NONE', #24965 ) ;
#3155=VERTEX_POINT ( 'NONE', #19437 ) ;
#3159=DIRECTION ( 'NONE',  ( 0.000000000000000000, -1.000000000000000000, 2.999999999999999839E-15 ) ) ;
#3161=EDGE_CURVE ( 'NONE', #22433, #9537, #7345, .T. ) ;
#3167=CIRCLE ( 'NONE', #5637, 0.5000000000000004441 ) ;
#3168=LINE ( 'NONE', #11040, #16121 ) ;
#3169=DIRECTION ( 'NONE',  ( 0.000000000000000000, 2.999999999999999839E-15, 1.000000000000000000 ) ) ;
#3170=VECTOR ( 'NONE', #9731, 1000.000000000000000 ) ;
#3192=DIRECTION ( 'NONE',  ( 1.000000000000000000, 0.000000000000000000, 0.000000000000000000 ) ) ;
#3194=VERTEX_POINT ( 'NONE', #9298 ) ;
#3207=ORIENTED_EDGE ( 'NONE', *, *, #7740, .F. ) ;
#3209=CARTESIAN_POINT ( 'NONE',  ( 32.81606138205700773, 35.44123852234597649, 68.30501292736990138 ) ) ;
#3211=CARTESIAN_POINT ( 'NONE',  ( 44.81606138205700063, 39.55420052130484265, 58.58767820587064534 ) ) ;
#3219=DIRECTION ( 'NONE',  ( 0.000000000000000000, -1.000000000000000000, 2.999999999999999839E-15 ) ) ;
#3220=ORIENTED_EDGE ( 'NONE', *, *, #17581, .T. ) ;
#3231=LINE ( 'NONE', #22439, #21691 ) ;
#3241=DIRECTION ( 'NONE',  ( -1.000000000000000000, 1.115179377413661005E-30, 3.717264591378870232E-16 ) ) ;
#3242=AXIS2_PLACEMENT_3D ( 'NONE', #3828, #11709, #1259 ) ;
#3244=CARTESIAN_POINT ( 'NONE',  ( 33.56606138205700773, -34.55876147765400219, 75.30501292737011454 ) ) ;
#3254=EDGE_CURVE ( 'NONE', #8848, #4816, #21251, .T. ) ;
#3255=EDGE_CURVE ( 'NONE', #2367, #6757, #7730, .T. ) ;
#3264=CARTESIAN_POINT ( 'NONE',  ( 39.31606138205700063, 42.19123852234599781, 75.30501292736987295 ) ) ;
#3265=FACE_OUTER_BOUND ( 'NONE', #16565, .T. ) ;
#3270=CARTESIAN_POINT ( 'NONE',  ( 44.81606138205700063, -22.55876147765401996, 68.80501292737008612 ) ) ;
#3284=EDGE_CURVE ( 'NONE', #25152, #10647, #5413, .T. ) ;
#3286=PLANE ( 'NONE',  #19042 ) ;
#3293=CYLINDRICAL_SURFACE ( 'NONE', #19734, 1.000000000000000888 ) ;
#3298=CARTESIAN_POINT ( 'NONE',  ( 40.31606138205700773, -31.05876147765400574, 73.55501292737010033 ) ) ;
#3317=EDGE_CURVE ( 'NONE', #16994, #4665, #1649, .T. ) ;
#3324=FACE_OUTER_BOUND ( 'NONE', #652, .T. ) ;
#3326=ORIENTED_EDGE ( 'NONE', *, *, #7846, .T. ) ;
#3336=DIRECTION ( 'NONE',  ( -1.000000000000000000, 0.000000000000000000, 0.000000000000000000 ) ) ;
#3341=EDGE_CURVE ( 'NONE', #4343, #20215, #16083, .T. ) ;
#3360=EDGE_LOOP ( 'NONE', ( #15024, #19497, #9144, #3504 ) ) ;
#3364=VECTOR ( 'NONE', #12666, 1000.000000000000000 ) ;
#3366=FACE_OUTER_BOUND ( 'NONE', #13790, .T. ) ;
#3378=FACE_OUTER_BOUND ( 'NONE', #3000, .T. ) ;
#3397=CARTESIAN_POINT ( 'NONE',  ( 43.06606138205700063, 41.44123852234599070, 73.55501292736987295 ) ) ;
#3399=EDGE_LOOP ( 'NONE', ( #3784, #21354, #17130, #15149 ) ) ;
#3411=EDGE_LOOP ( 'NONE', ( #23488, #7531, #177, #14835 ) ) ;
#3413=EDGE_LOOP ( 'NONE', ( #19615, #17036, #3971, #3094 ) ) ;
#3422=CIRCLE ( 'NONE', #6705, 1.000000000000000888 ) ;
#3448=AXIS2_PLACEMENT_3D ( 'NONE', #19213, #15732, #23195 ) ;
#3450=DIRECTION ( 'NONE',  ( 0.000000000000000000, 4.476705744456288765E-15, 1.000000000000000000 ) ) ;
#3462=AXIS2_PLACEMENT_3D ( 'NONE', #11467, #19304, #1774 ) ;
#3466=VERTEX_POINT ( 'NONE', #15831 ) ;
#3467=CARTESIAN_POINT ( 'NONE',  ( 41.31606138205687273, 33.19123852234595518, 61.30501292736990848 ) ) ;
#3468=DIRECTION ( 'NONE',  ( 0.000000000000000000, 1.000000000000000000, 0.000000000000000000 ) ) ;
#3470=ORIENTED_EDGE ( 'NONE', *, *, #9002, .F. ) ;
#3474=AXIS2_PLACEMENT_3D ( 'NONE', #7406, #20807, #21185 ) ;
#3480=LINE ( 'NONE', #1420, #359 ) ;
#3483=VERTEX_POINT ( 'NONE', #6051 ) ;
#3484=EDGE_CURVE ( 'NONE', #21718, #23642, #13907, .T. ) ;
#3487=EDGE_CURVE ( 'NONE', #4816, #16043, #2171, .T. ) ;
#3504=ORIENTED_EDGE ( 'NONE', *, *, #16814, .F. ) ;
#3507=VECTOR ( 'NONE', #24321, 1000.000000000000000 ) ;
#3539=ORIENTED_EDGE ( 'NONE', *, *, #20763, .F. ) ;
#3541=CARTESIAN_POINT ( 'NONE',  ( 31.81606138205700418, -34.55876147765400930, 73.30501292737011454 ) ) ;
#3551=ORIENTED_EDGE ( 'NONE', *, *, #14599, .F. ) ;
#3570=ORIENTED_EDGE ( 'NONE', *, *, #22873, .T. ) ;
#3572=DIRECTION ( 'NONE',  ( 0.000000000000000000, 1.000000000000000000, 0.000000000000000000 ) ) ;
#3574=ORIENTED_EDGE ( 'NONE', *, *, #16965, .F. ) ;
#3575=ADVANCED_FACE ( 'NONE', ( #18412 ), #6675, .F. ) ;
#3576=ORIENTED_EDGE ( 'NONE', *, *, #16976, .T. ) ;
#3579=FACE_OUTER_BOUND ( 'NONE', #2632, .T. ) ;
#3590=VECTOR ( 'NONE', #21544, 1000.000000000000000 ) ;
#3594=DIRECTION ( 'NONE',  ( 0.000000000000000000, -1.000000000000000000, 2.999999999999999839E-15 ) ) ;
#3604=ORIENTED_EDGE ( 'NONE', *, *, #12267, .F. ) ;
#3636=EDGE_LOOP ( 'NONE', ( #1444, #2774, #9496, #19580 ) ) ;
#3638=DIRECTION ( 'NONE',  ( -1.000000000000000000, 5.510910596163088391E-31, 1.836970198721029688E-16 ) ) ;
#3642=ORIENTED_EDGE ( 'NONE', *, *, #3284, .F. ) ;
#3649=PLANE ( 'NONE',  #1415 ) ;
#3652=EDGE_CURVE ( 'NONE', #3483, #64, #12743, .T. ) ;
#3654=EDGE_LOOP ( 'NONE', ( #4673, #23728, #13093, #24778 ) ) ;
#3660=DIRECTION ( 'NONE',  ( -1.000000000000000000, 5.510910596163088391E-31, 1.836970198721029688E-16 ) ) ;
#3670=EDGE_CURVE ( 'NONE', #5342, #13145, #17251, .T. ) ;
#3672=EDGE_LOOP ( 'NONE', ( #20762, #21747, #5918, #8628 ) ) ;
#3673=ORIENTED_EDGE ( 'NONE', *, *, #66, .F. ) ;
#3674=DIRECTION ( 'NONE',  ( 3.717264591378870232E-16, 3.115648231731786715E-15, 1.000000000000000000 ) ) ;
#3684=CARTESIAN_POINT ( 'NONE',  ( 44.81606138205700063, 41.44123852234599781, 75.30501292736987295 ) ) ;
#3689=CIRCLE ( 'NONE', #13154, 0.7500000000000006661 ) ;
#3694=FACE_OUTER_BOUND ( 'NONE', #8093, .T. ) ;
#3700=ADVANCED_FACE ( 'NONE', ( #24818, #19044 ), #25062, .F. ) ;
#3712=VERTEX_POINT ( 'NONE', #16185 ) ;
#3714=FACE_BOUND ( 'NONE', #15584, .T. ) ;
#3722=VECTOR ( 'NONE', #21598, 1000.000000000000000 ) ;
#3729=CYLINDRICAL_SURFACE ( 'NONE', #20555, 2.500000000000002220 ) ;
#3732=VERTEX_POINT ( 'NONE', #14139 ) ;
#3746=VECTOR ( 'NONE', #17871, 1000.000000000000000 ) ;
#3752=EDGE_CURVE ( 'NONE', #5864, #17161, #2432, .T. ) ;
#3774=EDGE_LOOP ( 'NONE', ( #21500, #4957, #18878, #15099, #18536, #11335, #278, #18169, #9610, #186, #20133, #5812 ) ) ;
#3783=AXIS2_PLACEMENT_3D ( 'NONE', #9531, #17375, #1894 ) ;
#3784=ORIENTED_EDGE ( 'NONE', *, *, #3255, .T. ) ;
#3787=CARTESIAN_POINT ( 'NONE',  ( 31.81606138205700418, 41.44123852234595518, 61.30501292736988006 ) ) ;
#3791=VERTEX_POINT ( 'NONE', #6153 ) ;
#3798=ORIENTED_EDGE ( 'NONE', *, *, #24971, .F. ) ;
#3820=ORIENTED_EDGE ( 'NONE', *, *, #10423, .F. ) ;
#3826=CYLINDRICAL_SURFACE ( 'NONE', #5656, 0.7500000000000006661 ) ;
#3828=CARTESIAN_POINT ( 'NONE',  ( 43.81606138205700063, -24.55876147765401285, 70.30501292737008612 ) ) ;
#3830=AXIS2_PLACEMENT_3D ( 'NONE', #14969, #5311, #14584 ) ;
#3842=AXIS2_PLACEMENT_3D ( 'NONE', #19111, #7256, #23464 ) ;
#3845=DIRECTION ( 'NONE',  ( 1.000000000000000000, 0.000000000000000000, 0.000000000000000000 ) ) ;
#3856=DIRECTION ( 'NONE',  ( 0.000000000000000000, 1.000000000000000000, 0.000000000000000000 ) ) ;
#3873=DIRECTION ( 'NONE',  ( -1.000000000000000000, 5.510910596163088391E-31, 1.836970198721029688E-16 ) ) ;
#3887=CARTESIAN_POINT ( 'NONE',  ( 44.81606138205700063, -34.55876147765400219, 74.30501292737011454 ) ) ;
#3888=AXIS2_PLACEMENT_3D ( 'NONE', #5596, #23232, #15884 ) ;
#3905=ORIENTED_EDGE ( 'NONE', *, *, #2203, .T. ) ;
#3911=ORIENTED_EDGE ( 'NONE', *, *, #4063, .F. ) ;
#3915=ORIENTED_EDGE ( 'NONE', *, *, #22950, .F. ) ;
#3929=CARTESIAN_POINT ( 'NONE',  ( 42.06606138205700063, 42.19123852234599781, 74.30501292736987295 ) ) ;
#3950=CARTESIAN_POINT ( 'NONE',  ( 43.06606138205700063, 41.44123852234599781, 75.30501292736987295 ) ) ;
#3951=LINE ( 'NONE', #21605, #16212 ) ;
#3957=DIRECTION ( 'NONE',  ( 0.000000000000000000, 1.000000000000000000, 0.000000000000000000 ) ) ;
#3961=VECTOR ( 'NONE', #2199, 1000.000000000000000 ) ;
#3971=ORIENTED_EDGE ( 'NONE', *, *, #2927, .T. ) ;
#3976=CARTESIAN_POINT ( 'NONE',  ( 40.31606138205700773, 42.19123852234599781, 74.30501292736987295 ) ) ;
#3981=EDGE_CURVE ( 'NONE', #2408, #16502, #16837, .T. ) ;
#3982=CARTESIAN_POINT ( 'NONE',  ( 31.81606138205700418, 38.19123852234599070, 72.05501292736988717 ) ) ;
#3992=CYLINDRICAL_SURFACE ( 'NONE', #24663, 0.5000000000000004441 ) ;
#4002=VECTOR ( 'NONE', #21853, 1000.000000000000000 ) ;
#4020=AXIS2_PLACEMENT_3D ( 'NONE', #9478, #5723, #24234 ) ;
#4027=ORIENTED_EDGE ( 'NONE', *, *, #24359, .F. ) ;
#4029=ORIENTED_EDGE ( 'NONE', *, *, #24971, .T. ) ;
#4034=ORIENTED_EDGE ( 'NONE', *, *, #22950, .T. ) ;
#4043=ORIENTED_EDGE ( 'NONE', *, *, #11729, .F. ) ;
#4045=ORIENTED_EDGE ( 'NONE', *, *, #21435, .F. ) ;
#4055=VERTEX_POINT ( 'NONE', #6794 ) ;
#4058=ORIENTED_EDGE ( 'NONE', *, *, #4137, .T. ) ;
#4062=AXIS2_PLACEMENT_3D ( 'NONE', #18888, #22368, #24409 ) ;
#4063=EDGE_CURVE ( 'NONE', #17824, #3140, #3689, .T. ) ;
#4074=ORIENTED_EDGE ( 'NONE', *, *, #11929, .T. ) ;
#4077=EDGE_LOOP ( 'NONE', ( #9685, #7046, #5534, #5512 ) ) ;
#4081=LINE ( 'NONE', #21978, #15298 ) ;
#4085=ORIENTED_EDGE ( 'NONE', *, *, #18873, .F. ) ;
#4089=FACE_OUTER_BOUND ( 'NONE', #12981, .T. ) ;
#4091=LINE ( 'NONE', #2393, #22535 ) ;
#4096=AXIS2_PLACEMENT_3D ( 'NONE', #1503, #23531, #5521 ) ;
#4100=EDGE_CURVE ( 'NONE', #2309, #7176, #13576, .T. ) ;
#4102=ORIENTED_EDGE ( 'NONE', *, *, #11819, .F. ) ;
#4106=CIRCLE ( 'NONE', #21359, 1.000000000000000888 ) ;
#4108=DIRECTION ( 'NONE',  ( 0.000000000000000000, 2.775557561562888984E-15, 1.000000000000000000 ) ) ;
#4128=CARTESIAN_POINT ( 'NONE',  ( 32.81606138205700773, -34.55876147765401640, 70.30501292737011454 ) ) ;
#4130=VERTEX_POINT ( 'NONE', #14893 ) ;
#4137=EDGE_CURVE ( 'NONE', #17161, #8796, #22628, .T. ) ;
#4141=ORIENTED_EDGE ( 'NONE', *, *, #4374, .T. ) ;
#4146=CARTESIAN_POINT ( 'NONE',  ( 40.81606138205700773, 37.44123852234599781, 75.30501292736990138 ) ) ;
#4149=AXIS2_PLACEMENT_3D ( 'NONE', #14931, #18796, #5151 ) ;
#4151=AXIS2_PLACEMENT_3D ( 'NONE', #18538, #14661, #7069 ) ;
#4162=ORIENTED_EDGE ( 'NONE', *, *, #6530, .F. ) ;
#4182=EDGE_CURVE ( 'NONE', #19667, #13053, #2448, .T. ) ;
#4187=AXIS2_PLACEMENT_3D ( 'NONE', #4274, #2197, #17935 ) ;
#4192=ORIENTED_EDGE ( 'NONE', *, *, #18873, .T. ) ;
#4194=FACE_OUTER_BOUND ( 'NONE', #13448, .T. ) ;
#4196=ADVANCED_FACE ( 'NONE', ( #14241 ), #14487, .T. ) ;
#4197=EDGE_CURVE ( 'NONE', #14420, #15888, #20972, .T. ) ;
#4199=VERTEX_POINT ( 'NONE', #17982 ) ;
#4201=DIRECTION ( 'NONE',  ( -3.491481338843135327E-15, 1.000000000000000000, -2.999999999999999839E-15 ) ) ;
#4210=CARTESIAN_POINT ( 'NONE',  ( 43.81606138205700063, -38.55876147765404482, 61.30501292737012164 ) ) ;
#4216=CARTESIAN_POINT ( 'NONE',  ( 43.81606138205700063, -34.55876147765404482, 61.30501292737010743 ) ) ;
#4237=VECTOR ( 'NONE', #22258, 1000.000000000000000 ) ;
#4250=CARTESIAN_POINT ( 'NONE',  ( 31.81606138205700418, 38.19123852234599070, 73.05501292736988717 ) ) ;
#4257=ADVANCED_FACE ( 'NONE', ( #20409 ), #8444, .F. ) ;
#4259=CARTESIAN_POINT ( 'NONE',  ( 38.31606138205687984, 42.19123852234599781, 75.30501292736987295 ) ) ;
#4267=CARTESIAN_POINT ( 'NONE',  ( 32.81606138205700773, -34.55876147765400930, 73.55501292737011454 ) ) ;
#4270=CARTESIAN_POINT ( 'NONE',  ( 36.31606138205700063, -29.30876147765400574, 73.55501292737010033 ) ) ;
#4274=CARTESIAN_POINT ( 'NONE',  ( 43.06606138205700063, 41.44123852234599070, 73.55501292736987295 ) ) ;
#4276=CARTESIAN_POINT ( 'NONE',  ( 43.06606138205700063, -34.55876147765400219, 74.30501292737011454 ) ) ;
#4278=AXIS2_PLACEMENT_3D ( 'NONE', #16749, #6459, #14444 ) ;
#4290=DIRECTION ( 'NONE',  ( -1.000000000000000000, 5.204170427930415223E-30, 1.734723475976805122E-15 ) ) ;
#4316=SHAPE_REPRESENTATION_RELATIONSHIP ( 'NONE' , 'NONE' ,  #7525, #21819 ) ;
#4318=EDGE_CURVE ( 'NONE', #15787, #23679, #19912, .T. ) ;
#4330=FACE_OUTER_BOUND ( 'NONE', #11440, .T. ) ;
#4336=CARTESIAN_POINT ( 'NONE',  ( 32.81606138205700773, 38.19123852234599070, 72.05501292736988717 ) ) ;
#4338=DIRECTION ( 'NONE',  ( 0.000000000000000000, -1.000000000000000000, 2.999999999999999839E-15 ) ) ;
#4339=CARTESIAN_POINT ( 'NONE',  ( 43.06606138205700063, 41.44123852234595518, 61.30501292736988006 ) ) ;
#4342=DIRECTION ( 'NONE',  ( 0.000000000000000000, 2.999999999999999839E-15, 1.000000000000000000 ) ) ;
#4343=VERTEX_POINT ( 'NONE', #7009 ) ;
#4361=EDGE_CURVE ( 'NONE', #13874, #22091, #13202, .T. ) ;
#4374=EDGE_CURVE ( 'NONE', #7542, #13262, #24629, .T. ) ;
#4385=PRODUCT_DEFINITION_CONTEXT ( 'detailed design', #14412, 'design' ) ;
#4400=CARTESIAN_POINT ( 'NONE',  ( 40.81606138205700773, 37.44123852234599781, 74.30501292736988717 ) ) ;
#4409=VECTOR ( 'NONE', #7425, 1000.000000000000000 ) ;
#4426=DIRECTION ( 'NONE',  ( 1.734723475976805122E-15, 2.999999999999999839E-15, 1.000000000000000000 ) ) ;
#4435=LINE ( 'NONE', #293, #7566 ) ;
#4438=( NAMED_UNIT ( * ) SI_UNIT ( $, .STERADIAN. ) SOLID_ANGLE_UNIT ( ) );
#4441=PLANE ( 'NONE',  #1231 ) ;
#4444=VERTEX_POINT ( 'NONE', #9088 ) ;
#4446=ORIENTED_EDGE ( 'NONE', *, *, #23269, .T. ) ;
#4457=DIRECTION ( 'NONE',  ( -1.000000000000000000, 0.000000000000000000, 0.000000000000000000 ) ) ;
#4459=EDGE_LOOP ( 'NONE', ( #4141, #879, #5571, #13289, #17921, #7428, #10034, #16834, #22724, #1055, #6289 ) ) ;
#4462=EDGE_CURVE ( 'NONE', #1877, #5235, #16931, .T. ) ;
#4464=DIRECTION ( 'NONE',  ( 0.000000000000000000, 1.000000000000000000, -2.999999999999999839E-15 ) ) ;
#4467=CARTESIAN_POINT ( 'NONE',  ( 44.81606138205700063, 35.44123852234597649, 68.30501292736990138 ) ) ;
#4468=VERTEX_POINT ( 'NONE', #23097 ) ;
#4470=EDGE_LOOP ( 'NONE', ( #221, #7971, #22462, #16093 ) ) ;
#4471=CARTESIAN_POINT ( 'NONE',  ( 40.31606138205700773, 43.19123852234596939, 65.30501292736988717 ) ) ;
#4489=DIRECTION ( 'NONE',  ( 1.000000000000000000, 0.000000000000000000, 0.000000000000000000 ) ) ;
#4497=CARTESIAN_POINT ( 'NONE',  ( 43.06606138205700063, -38.55876147765401640, 70.30501292737012875 ) ) ;
#4507=ORIENTED_EDGE ( 'NONE', *, *, #13250, .F. ) ;
#4514=CARTESIAN_POINT ( 'NONE',  ( 38.31606138205700063, 42.51966564709218233, 71.30501292737018559 ) ) ;
#4523=CARTESIAN_POINT ( 'NONE',  ( 38.31606138205700063, -30.30876147765399864, 75.30501292736995822 ) ) ;
#4525=CARTESIAN_POINT ( 'NONE',  ( 32.81606138205700773, 28.12806996228107081, 65.30501292736992980 ) ) ;
#4530=AXIS2_PLACEMENT_3D ( 'NONE', #157, #15623, #25 ) ;
#4559=CYLINDRICAL_SURFACE ( 'NONE', #20756, 1.000000000000000888 ) ;
#4562=DIRECTION ( 'NONE',  ( 1.000000000000000000, -1.011922027653136605E-30, -3.373073425510455500E-16 ) ) ;
#4564=DIRECTION ( 'NONE',  ( 1.000000000000000000, 0.000000000000000000, 0.000000000000000000 ) ) ;
#4571=CARTESIAN_POINT ( 'NONE',  ( 35.81606138205700063, 41.44123852234599781, 74.30501292736987295 ) ) ;
#4575=CARTESIAN_POINT ( 'NONE',  ( 36.31606138205700063, -29.30876147765400574, 73.55501292737010033 ) ) ;
#4577=ADVANCED_FACE ( 'NONE', ( #9838 ), #5839, .T. ) ;
#4579=ORIENTED_EDGE ( 'NONE', *, *, #24838, .T. ) ;
#4581=DIRECTION ( 'NONE',  ( -1.000000000000000000, 0.000000000000000000, 0.000000000000000000 ) ) ;
#4586=ORIENTED_EDGE ( 'NONE', *, *, #22066, .F. ) ;
#4589=VERTEX_POINT ( 'NONE', #1698 ) ;
#4599=PLANE ( 'NONE',  #9606 ) ;
#4620=CYLINDRICAL_SURFACE ( 'NONE', #18917, 1.000000000000000888 ) ;
#4636=CARTESIAN_POINT ( 'NONE',  ( 40.81606138205700773, -31.05876147765399864, 74.30501292737010033 ) ) ;
#4647=DIRECTION ( 'NONE',  ( 1.000000000000000000, 0.000000000000000000, 0.000000000000000000 ) ) ;
#4660=ORIENTED_EDGE ( 'NONE', *, *, #16719, .F. ) ;
#4662=PLANE ( 'NONE',  #12646 ) ;
#4665=VERTEX_POINT ( 'NONE', #1572 ) ;
#4667=ORIENTED_EDGE ( 'NONE', *, *, #14980, .F. ) ;
#4673=ORIENTED_EDGE ( 'NONE', *, *, #18785, .F. ) ;
#4679=CARTESIAN_POINT ( 'NONE',  ( 31.81606138205700418, -36.55876147765400930, 73.30501292737011454 ) ) ;
#4690=ADVANCED_FACE ( 'NONE', ( #531 ), #10216, .F. ) ;
#4712=EDGE_CURVE ( 'NONE', #6796, #6622, #18079, .T. ) ;
#4719=VERTEX_POINT ( 'NONE', #6473 ) ;
#4725=AXIS2_PLACEMENT_3D ( 'NONE', #16685, #18875, #22984 ) ;
#4728=DIRECTION ( 'NONE',  ( 3.965082230804126670E-15, 1.000000000000000000, -3.965082230804126670E-15 ) ) ;
#4729=CARTESIAN_POINT ( 'NONE',  ( 44.81606138205700063, -34.55876147765401640, 70.30501292737011454 ) ) ;
#4732=EDGE_LOOP ( 'NONE', ( #17866, #21021, #20029, #20843 ) ) ;
#4734=CARTESIAN_POINT ( 'NONE',  ( 44.81606138205700063, 35.44123852234597649, 67.80501292736990138 ) ) ;
#4737=ORIENTED_EDGE ( 'NONE', *, *, #2778, .T. ) ;
#4750=ORIENTED_EDGE ( 'NONE', *, *, #7200, .T. ) ;
#4760=ORIENTED_EDGE ( 'NONE', *, *, #19396, .F. ) ;
#4764=ORIENTED_EDGE ( 'NONE', *, *, #5065, .F. ) ;
#4800=DIRECTION ( 'NONE',  ( 0.000000000000000000, 1.000000000000000000, -2.999999999999999839E-15 ) ) ;
#4805=FACE_OUTER_BOUND ( 'NONE', #2180, .T. ) ;
#4808=DIRECTION ( 'NONE',  ( 1.734723475976805122E-15, 2.999999999999999839E-15, 1.000000000000000000 ) ) ;
#4815=ORIENTED_EDGE ( 'NONE', *, *, #5363, .F. ) ;
#4816=VERTEX_POINT ( 'NONE', #22309 ) ;
#4830=LINE ( 'NONE', #20173, #19105 ) ;
#4836=EDGE_CURVE ( 'NONE', #13311, #16934, #15998, .T. ) ;
#4851=CARTESIAN_POINT ( 'NONE',  ( 40.31606138205700773, -30.30876147765401996, 69.30501292737010033 ) ) ;
#4856=CARTESIAN_POINT ( 'NONE',  ( 43.06606138205700063, 41.44123852234599070, 73.55501292736987295 ) ) ;
#4885=CARTESIAN_POINT ( 'NONE',  ( 38.31606138205700063, 38.69123852234598360, 70.30501292737018559 ) ) ;
#4890=CARTESIAN_POINT ( 'NONE',  ( 43.81606138205700063, 41.44123852234599070, 73.55501292736987295 ) ) ;
#4894=FACE_OUTER_BOUND ( 'NONE', #7906, .T. ) ;
#4899=AXIS2_PLACEMENT_3D ( 'NONE', #1645, #19694, #25216 ) ;
#4909=EDGE_CURVE ( 'NONE', #15787, #12138, #11978, .T. ) ;
#4916=ORIENTED_EDGE ( 'NONE', *, *, #2727, .T. ) ;
#4924=FACE_OUTER_BOUND ( 'NONE', #3399, .T. ) ;
#4928=LINE ( 'NONE', #2979, #7917 ) ;
#4933=CARTESIAN_POINT ( 'NONE',  ( 32.81606138205700773, 41.44123852234596939, 66.30501292736988717 ) ) ;
#4935=VERTEX_POINT ( 'NONE', #6846 ) ;
#4940=DIRECTION ( 'NONE',  ( -1.000000000000000000, 0.000000000000000000, 0.000000000000000000 ) ) ;
#4942=DIRECTION ( 'NONE',  ( 1.836970198721029688E-16, 2.999999999999999839E-15, 1.000000000000000000 ) ) ;
#4952=VECTOR ( 'NONE', #21872, 1000.000000000000000 ) ;
#4957=ORIENTED_EDGE ( 'NONE', *, *, #9293, .T. ) ;
#4965=CARTESIAN_POINT ( 'NONE',  ( 38.31606138205700063, -29.30876147765401285, 70.30501292737010033 ) ) ;
#4973=DIRECTION ( 'NONE',  ( 0.000000000000000000, -1.000000000000000000, 2.999999999999999839E-15 ) ) ;
#4977=DIRECTION ( 'NONE',  ( -1.000000000000000000, 1.115179377413661005E-30, 3.717264591378870232E-16 ) ) ;
#4983=ORIENTED_EDGE ( 'NONE', *, *, #20373, .T. ) ;
#5004=ORIENTED_EDGE ( 'NONE', *, *, #10423, .T. ) ;
#5006=LINE ( 'NONE', #17242, #2043 ) ;
#5008=CARTESIAN_POINT ( 'NONE',  ( 33.56606138205700773, 43.19123852234595518, 61.30501292736988006 ) ) ;
#5010=EDGE_CURVE ( 'NONE', #6622, #17440, #23034, .T. ) ;
#5013=ADVANCED_FACE ( 'NONE', ( #11365, #9558 ), #21525, .F. ) ;
#5019=FACE_OUTER_BOUND ( 'NONE', #22381, .T. ) ;
#5023=VERTEX_POINT ( 'NONE', #21265 ) ;
#5050=AXIS2_PLACEMENT_3D ( 'NONE', #22514, #2794, #11191 ) ;
#5061=DIRECTION ( 'NONE',  ( 0.000000000000000000, -2.999999999999999839E-15, -1.000000000000000000 ) ) ;
#5064=EDGE_LOOP ( 'NONE', ( #11245, #7678, #7007, #22427 ) ) ;
#5065=EDGE_CURVE ( 'NONE', #14420, #19848, #5939, .T. ) ;
#5066=CARTESIAN_POINT ( 'NONE',  ( 43.06606138205700063, 42.19123852234595518, 61.30501292736988006 ) ) ;
#5081=ORIENTED_EDGE ( 'NONE', *, *, #25086, .T. ) ;
#5093=EDGE_LOOP ( 'NONE', ( #5978, #2781 ) ) ;
#5103=EDGE_CURVE ( 'NONE', #1244, #13733, #5813, .T. ) ;
#5110=CARTESIAN_POINT ( 'NONE',  ( 40.31606138205700773, 39.69123852234599070, 73.55501292736988717 ) ) ;
#5111=ORIENTED_EDGE ( 'NONE', *, *, #6671, .T. ) ;
#5114=CARTESIAN_POINT ( 'NONE',  ( 39.31606138205700063, 42.19123852234596939, 66.30501292736988717 ) ) ;
#5115=CARTESIAN_POINT ( 'NONE',  ( 44.81606138205700063, -22.55876147765401996, 68.80501292737008612 ) ) ;
#5126=ORIENTED_EDGE ( 'NONE', *, *, #18690, .T. ) ;
#5151=DIRECTION ( 'NONE',  ( -1.000000000000000000, 0.000000000000000000, 0.000000000000000000 ) ) ;
#5153=LINE ( 'NONE', #8897, #3507 ) ;
#5157=EDGE_CURVE ( 'NONE', #7176, #4719, #13297, .T. ) ;
#5159=DIRECTION ( 'NONE',  ( 0.000000000000000000, -3.469446951953611033E-15, -1.000000000000000000 ) ) ;
#5165=EDGE_CURVE ( 'NONE', #4816, #13486, #17296, .T. ) ;
#5176=EDGE_CURVE ( 'NONE', #15661, #12889, #19344, .T. ) ;
#5178=LINE ( 'NONE', #24726, #23399 ) ;
#5203=DIRECTION ( 'NONE',  ( -1.000000000000000000, 0.000000000000000000, 0.000000000000000000 ) ) ;
#5223=ORIENTED_EDGE ( 'NONE', *, *, #20043, .F. ) ;
#5235=VERTEX_POINT ( 'NONE', #6564 ) ;
#5241=CARTESIAN_POINT ( 'NONE',  ( 43.06606138205700063, 41.44123852234599070, 73.55501292736987295 ) ) ;
#5247=VERTEX_POINT ( 'NONE', #12383 ) ;
#5256=EDGE_CURVE ( 'NONE', #16707, #9905, #8122, .T. ) ;
#5258=VECTOR ( 'NONE', #5681, 1000.000000000000000 ) ;
#5261=DIRECTION ( 'NONE',  ( 9.027796614315171564E-31, 1.000000000000000000, 1.163336342344340343E-15 ) ) ;
#5263=PLANE ( 'NONE',  #4096 ) ;
#5282=ADVANCED_FACE ( 'NONE', ( #18175 ), #14048, .T. ) ;
#5290=DIRECTION ( 'NONE',  ( -1.836970198721029688E-16, -2.999999999999999839E-15, -1.000000000000000000 ) ) ;
#5292=EDGE_LOOP ( 'NONE', ( #15250, #1263, #620, #16960 ) ) ;
#5303=DIRECTION ( 'NONE',  ( 0.000000000000000000, 2.775557561562888984E-15, 1.000000000000000000 ) ) ;
#5309=ORIENTED_EDGE ( 'NONE', *, *, #21754, .T. ) ;
#5311=DIRECTION ( 'NONE',  ( 0.000000000000000000, 2.999999999999999839E-15, 1.000000000000000000 ) ) ;
#5314=CIRCLE ( 'NONE', #18061, 2.000000000000001776 ) ;
#5317=CARTESIAN_POINT ( 'NONE',  ( 36.31606138205700063, 37.94123852234599781, 74.30501292736988717 ) ) ;
#5340=AXIS2_PLACEMENT_3D ( 'NONE', #18358, #24385, #10505 ) ;
#5342=VERTEX_POINT ( 'NONE', #23946 ) ;
#5353=AXIS2_PLACEMENT_3D ( 'NONE', #17531, #19577, #6056 ) ;
#5363=EDGE_CURVE ( 'NONE', #22433, #8848, #18671, .T. ) ;
#5368=DIRECTION ( 'NONE',  ( 0.000000000000000000, -1.000000000000000000, 2.999999999999999839E-15 ) ) ;
#5370=VERTEX_POINT ( 'NONE', #4885 ) ;
#5372=CARTESIAN_POINT ( 'NONE',  ( 44.81606138205700063, -36.55876147765400930, 73.30501292737011454 ) ) ;
#5381=ORIENTED_EDGE ( 'NONE', *, *, #10858, .F. ) ;
#5389=EDGE_CURVE ( 'NONE', #10647, #11848, #9021, .T. ) ;
#5406=LINE ( 'NONE', #7599, #8403 ) ;
#5411=DIRECTION ( 'NONE',  ( 1.734723475976804876E-16, -1.163336342344340343E-15, 1.000000000000000000 ) ) ;
#5412=AXIS2_PLACEMENT_3D ( 'NONE', #4339, #12201, #20040 ) ;
#5413=LINE ( 'NONE', #5543, #7357 ) ;
#5419=CARTESIAN_POINT ( 'NONE',  ( 32.81606138205700773, -38.55876147765400219, 75.30501292737012875 ) ) ;
#5432=ORIENTED_EDGE ( 'NONE', *, *, #6671, .F. ) ;
#5434=PLANE ( 'NONE',  #1776 ) ;
#5440=DIRECTION ( 'NONE',  ( 0.000000000000000000, -6.938893903907222067E-15, 1.000000000000000000 ) ) ;
#5443=CARTESIAN_POINT ( 'NONE',  ( 43.81606138205700063, 41.44123852234595518, 61.30501292736988006 ) ) ;
#5450=VECTOR ( 'NONE', #4338, 1000.000000000000000 ) ;
#5453=VECTOR ( 'NONE', #22391, 1000.000000000000000 ) ;
#5462=ORIENTED_EDGE ( 'NONE', *, *, #12289, .T. ) ;
#5467=CARTESIAN_POINT ( 'NONE',  ( 31.81606138205700418, 35.44123852234597649, 67.80501292736990138 ) ) ;
#5472=DIRECTION ( 'NONE',  ( -3.965082230804126670E-15, 1.000000000000000000, 0.000000000000000000 ) ) ;
#5479=VECTOR ( 'NONE', #18003, 1000.000000000000000 ) ;
#5489=CARTESIAN_POINT ( 'NONE',  ( 43.81606138205700063, 35.95440708241085304, 62.30501292736990138 ) ) ;
#5494=ADVANCED_FACE ( 'NONE', ( #6687 ), #10945, .F. ) ;
#5505=CARTESIAN_POINT ( 'NONE',  ( 36.31606138205700063, 37.94123852234599070, 73.55501292736988717 ) ) ;
#5512=ORIENTED_EDGE ( 'NONE', *, *, #11569, .F. ) ;
#5518=DIRECTION ( 'NONE',  ( 0.000000000000000000, 2.999999999999999839E-15, 1.000000000000000000 ) ) ;
#5521=DIRECTION ( 'NONE',  ( 3.540251991789399939E-16, 2.999999999999999839E-15, 1.000000000000000000 ) ) ;
#5522=VERTEX_POINT ( 'NONE', #23260 ) ;
#5524=CARTESIAN_POINT ( 'NONE',  ( 33.56606138205700773, 41.44123852234599070, 73.55501292736987295 ) ) ;
#5526=ORIENTED_EDGE ( 'NONE', *, *, #19837, .F. ) ;
#5534=ORIENTED_EDGE ( 'NONE', *, *, #18690, .F. ) ;
#5538=ORIENTED_EDGE ( 'NONE', *, *, #5389, .T. ) ;
#5543=CARTESIAN_POINT ( 'NONE',  ( 35.81606138205700063, -24.05876147765399864, 75.30501292737008612 ) ) ;
#5548=DIRECTION ( 'NONE',  ( 0.000000000000000000, -1.000000000000000000, 2.999999999999999839E-15 ) ) ;
#5560=ADVANCED_FACE ( 'NONE', ( #16470 ), #19533, .T. ) ;
#5571=ORIENTED_EDGE ( 'NONE', *, *, #13684, .F. ) ;
#5575=VECTOR ( 'NONE', #6692, 1000.000000000000000 ) ;
#5596=CARTESIAN_POINT ( 'NONE',  ( 38.31606138205700063, -29.30876147765400930, 71.30501292737010033 ) ) ;
#5602=CARTESIAN_POINT ( 'NONE',  ( 44.81606138205700063, 41.44123852234599070, 73.55501292736987295 ) ) ;
#5607=DIRECTION ( 'NONE',  ( -4.336808689942020201E-16, -2.999999999999999839E-15, -1.000000000000000000 ) ) ;
#5610=ORIENTED_EDGE ( 'NONE', *, *, #15972, .T. ) ;
#5613=EDGE_LOOP ( 'NONE', ( #19666, #7306, #10537, #23116 ) ) ;
#5614=CARTESIAN_POINT ( 'NONE',  ( 44.81606138205700063, 1.441238522345976714, 67.80501292737001506 ) ) ;
#5621=DIRECTION ( 'NONE',  ( 1.000000000000000000, -6.938893903907222067E-15, 0.000000000000000000 ) ) ;
#5624=FACE_OUTER_BOUND ( 'NONE', #7098, .T. ) ;
#5630=ORIENTED_EDGE ( 'NONE', *, *, #9002, .T. ) ;
#5634=CARTESIAN_POINT ( 'NONE',  ( 31.81606138205700418, -24.55876147765401285, 70.30501292737008612 ) ) ;
#5637=AXIS2_PLACEMENT_3D ( 'NONE', #4467, #6268, #8459 ) ;
#5642=VERTEX_POINT ( 'NONE', #316 ) ;
#5647=EDGE_CURVE ( 'NONE', #17700, #4468, #12071, .T. ) ;
#5649=ORIENTED_EDGE ( 'NONE', *, *, #22948, .T. ) ;
#5651=CARTESIAN_POINT ( 'NONE',  ( 33.56606138205700773, 41.44123852234599781, 75.30501292736988717 ) ) ;
#5656=AXIS2_PLACEMENT_3D ( 'NONE', #207, #6277, #3957 ) ;
#5658=FACE_OUTER_BOUND ( 'NONE', #8760, .T. ) ;
#5659=EDGE_CURVE ( 'NONE', #9093, #13053, #25312, .T. ) ;
#5668=DIRECTION ( 'NONE',  ( -1.000000000000000000, 0.000000000000000000, 0.000000000000000000 ) ) ;
#5670=VECTOR ( 'NONE', #12137, 1000.000000000000000 ) ;
#5681=DIRECTION ( 'NONE',  ( -1.000000000000000000, 5.204170427930413997E-31, 1.734723475976804876E-16 ) ) ;
#5684=DIRECTION ( 'NONE',  ( 1.836970198721029688E-16, 2.999999999999999839E-15, 1.000000000000000000 ) ) ;
#5689=CARTESIAN_POINT ( 'NONE',  ( 31.81606138205700418, 38.19123852234599070, 72.05501292736988717 ) ) ;
#5698=( GEOMETRIC_REPRESENTATION_CONTEXT ( 3 ) GLOBAL_UNCERTAINTY_ASSIGNED_CONTEXT ( ( #685 ) ) GLOBAL_UNIT_ASSIGNED_CONTEXT ( ( #25478, #17647, #13522 ) ) REPRESENTATION_CONTEXT ( 'NONE', 'WORKASPACE' ) );
#5702=EDGE_CURVE ( 'NONE', #6796, #14420, #8073, .T. ) ;
#5711=CARTESIAN_POINT ( 'NONE',  ( 44.81606138205700063, 35.44123852234597649, 68.80501292736990138 ) ) ;
#5717=ADVANCED_FACE ( 'NONE', ( #17734 ), #8195, .T. ) ;
#5723=DIRECTION ( 'NONE',  ( 1.000000000000000000, 0.000000000000000000, 0.000000000000000000 ) ) ;
#5724=ORIENTED_EDGE ( 'NONE', *, *, #3652, .F. ) ;
#5725=VECTOR ( 'NONE', #19964, 1000.000000000000000 ) ;
#5733=EDGE_LOOP ( 'NONE', ( #8462, #4043, #17220, #25215 ) ) ;
#5736=DIRECTION ( 'NONE',  ( -2.120312145707929538E-16, 0.8213699656732942334, -0.5703958094953462954 ) ) ;
#5738=AXIS2_PLACEMENT_3D ( 'NONE', #19549, #10023, #18008 ) ;
#5743=PLANE ( 'NONE',  #9374 ) ;
#5750=EDGE_CURVE ( 'NONE', #16702, #5882, #443, .T. ) ;
#5752=ORIENTED_EDGE ( 'NONE', *, *, #3255, .F. ) ;
#5755=VECTOR ( 'NONE', #21960, 1000.000000000000000 ) ;
#5763=FACE_OUTER_BOUND ( 'NONE', #5064, .T. ) ;
#5771=EDGE_CURVE ( 'NONE', #19498, #5247, #20197, .T. ) ;
#5798=AXIS2_PLACEMENT_3D ( 'NONE', #9249, #15022, #22878 ) ;
#5799=EDGE_CURVE ( 'NONE', #9870, #24731, #12199, .T. ) ;
#5804=DIRECTION ( 'NONE',  ( -1.000000000000000000, 1.678764654171101651E-30, 5.595882180570339263E-16 ) ) ;
#5807=ORIENTED_EDGE ( 'NONE', *, *, #6965, .T. ) ;
#5812=ORIENTED_EDGE ( 'NONE', *, *, #20014, .T. ) ;
#5813=LINE ( 'NONE', #17155, #8244 ) ;
#5818=DIRECTION ( 'NONE',  ( 1.000000000000000000, 0.000000000000000000, 0.000000000000000000 ) ) ;
#5826=CARTESIAN_POINT ( 'NONE',  ( 35.81606138205700063, 37.44123852234599781, 75.30501292736990138 ) ) ;
#5839=PLANE ( 'NONE',  #4530 ) ;
#5845=PLANE ( 'NONE',  #14536 ) ;
#5854=CIRCLE ( 'NONE', #7484, 1.000000000000000888 ) ;
#5861=CIRCLE ( 'NONE', #16526, 0.5000000000000004441 ) ;
#5863=CYLINDRICAL_SURFACE ( 'NONE', #8364, 4.000000000000003553 ) ;
#5864=VERTEX_POINT ( 'NONE', #10639 ) ;
#5881=CARTESIAN_POINT ( 'NONE',  ( 32.81606138205700773, 35.44123852234597649, 68.80501292736990138 ) ) ;
#5882=VERTEX_POINT ( 'NONE', #14618 ) ;
#5883=CARTESIAN_POINT ( 'NONE',  ( 43.81606138205700063, 41.44123852234599070, 73.05501292736987295 ) ) ;
#5894=VECTOR ( 'NONE', #3638, 1000.000000000000000 ) ;
#5895=DIRECTION ( 'NONE',  ( 0.000000000000000000, 2.999999999999999839E-15, 1.000000000000000000 ) ) ;
#5904=DIRECTION ( 'NONE',  ( -1.000000000000000000, 0.000000000000000000, 0.000000000000000000 ) ) ;
#5909=VERTEX_POINT ( 'NONE', #13208 ) ;
#5910=DIRECTION ( 'NONE',  ( -1.000000000000000000, 1.040834085586084551E-30, 3.469446951953615175E-16 ) ) ;
#5918=ORIENTED_EDGE ( 'NONE', *, *, #19977, .F. ) ;
#5919=PLANE ( 'NONE',  #20095 ) ;
#5921=VECTOR ( 'NONE', #4800, 1000.000000000000000 ) ;
#5922=FACE_OUTER_BOUND ( 'NONE', #9575, .T. ) ;
#5924=EDGE_CURVE ( 'NONE', #20215, #13311, #3048, .T. ) ;
#5931=AXIS2_PLACEMENT_3D ( 'NONE', #23290, #21123, #3468 ) ;
#5939=LINE ( 'NONE', #9811, #811 ) ;
#5942=CYLINDRICAL_SURFACE ( 'NONE', #11871, 1.000000000000000888 ) ;
#5948=EDGE_CURVE ( 'NONE', #11106, #12188, #19927, .T. ) ;
#5949=CIRCLE ( 'NONE', #10050, 0.7500000000000006661 ) ;
#5951=EDGE_CURVE ( 'NONE', #20177, #17565, #11012, .T. ) ;
#5972=LINE ( 'NONE', #21297, #24381 ) ;
#5978=ORIENTED_EDGE ( 'NONE', *, *, #13903, .F. ) ;
#5994=DIRECTION ( 'NONE',  ( 1.000000000000000000, -1.115179377413661005E-30, -3.717264591378870232E-16 ) ) ;
#5999=ORIENTED_EDGE ( 'NONE', *, *, #21334, .F. ) ;
#6018=ORIENTED_EDGE ( 'NONE', *, *, #3254, .T. ) ;
#6022=FACE_OUTER_BOUND ( 'NONE', #4459, .T. ) ;
#6032=EDGE_CURVE ( 'NONE', #13165, #14570, #13077, .T. ) ;
#6038=CARTESIAN_POINT ( 'NONE',  ( 31.81606138205700418, -34.55876147765401640, 70.30501292737011454 ) ) ;
#6042=EDGE_CURVE ( 'NONE', #18207, #14131, #11658, .T. ) ;
#6051=CARTESIAN_POINT ( 'NONE',  ( 43.81606138205700063, -24.55876147765400574, 72.80501292737008612 ) ) ;
#6053=DIRECTION ( 'NONE',  ( -9.027796614315171564E-31, -1.000000000000000000, -1.163336342344335610E-15 ) ) ;
#6055=ORIENTED_EDGE ( 'NONE', *, *, #23872, .T. ) ;
#6056=DIRECTION ( 'NONE',  ( 0.000000000000000000, -4.625929269271481378E-15, -1.000000000000000000 ) ) ;
#6058=ORIENTED_EDGE ( 'NONE', *, *, #5659, .T. ) ;
#6066=VECTOR ( 'NONE', #18845, 1000.000000000000000 ) ;
#6070=PLANE ( 'NONE',  #6396 ) ;
#6077=LINE ( 'NONE', #3887, #22415 ) ;
#6085=VECTOR ( 'NONE', #22776, 1000.000000000000000 ) ;
#6089=ADVANCED_FACE ( 'NONE', ( #21684 ), #1960, .T. ) ;
#6092=ORIENTED_EDGE ( 'NONE', *, *, #15709, .F. ) ;
#6104=DIRECTION ( 'NONE',  ( 2.312964634635740294E-15, 2.999999999999999839E-15, 1.000000000000000000 ) ) ;
#6107=ORIENTED_EDGE ( 'NONE', *, *, #23872, .F. ) ;
#6110=DIRECTION ( 'NONE',  ( -1.000000000000000000, 1.040834085586084551E-30, 3.469446951953615175E-16 ) ) ;
#6117=LINE ( 'NONE', #13977, #22993 ) ;
#6124=ORIENTED_EDGE ( 'NONE', *, *, #6702, .T. ) ;
#6126=VERTEX_POINT ( 'NONE', #17701 ) ;
#6127=ORIENTED_EDGE ( 'NONE', *, *, #13988, .F. ) ;
#6128=DIRECTION ( 'NONE',  ( 1.000000000000000000, 0.000000000000000000, 0.000000000000000000 ) ) ;
#6135=CARTESIAN_POINT ( 'NONE',  ( 37.31606138205700063, 43.19123852234596939, 66.30501292736988717 ) ) ;
#6139=AXIS2_PLACEMENT_3D ( 'NONE', #24065, #14038, #10557 ) ;
#6144=AXIS2_PLACEMENT_3D ( 'NONE', #12895, #18555, #18805 ) ;
#6153=CARTESIAN_POINT ( 'NONE',  ( 44.81606138205700063, -36.55876147765400930, 73.30501292737011454 ) ) ;
#6158=ORIENTED_EDGE ( 'NONE', *, *, #10827, .T. ) ;
#6164=LINE ( 'NONE', #15558, #2128 ) ;
#6170=EDGE_CURVE ( 'NONE', #14470, #20177, #5949, .T. ) ;
#6173=DIRECTION ( 'NONE',  ( 1.000000000000000000, 0.000000000000000000, 0.000000000000000000 ) ) ;
#6180=DIRECTION ( 'NONE',  ( 0.000000000000000000, -1.000000000000000000, 2.999999999999999839E-15 ) ) ;
#6197=FACE_OUTER_BOUND ( 'NONE', #18252, .T. ) ;
#6200=DIRECTION ( 'NONE',  ( 0.000000000000000000, 3.469446951953611033E-15, 1.000000000000000000 ) ) ;
#6222=DIRECTION ( 'NONE',  ( 3.540251991789399939E-16, 2.999999999999999839E-15, 1.000000000000000000 ) ) ;
#6224=AXIS2_PLACEMENT_3D ( 'NONE', #3298, #14767, #22624 ) ;
#6226=EDGE_LOOP ( 'NONE', ( #13860, #15124, #4034, #4045 ) ) ;
#6240=DIRECTION ( 'NONE',  ( 0.000000000000000000, -2.913263826201159484E-15, -1.000000000000000000 ) ) ;
#6243=ADVANCED_FACE ( 'NONE', ( #537 ), #18456, .F. ) ;
#6247=ORIENTED_EDGE ( 'NONE', *, *, #7536, .T. ) ;
#6251=DIRECTION ( 'NONE',  ( -1.000000000000000000, 1.115179377413661005E-30, 3.717264591378870232E-16 ) ) ;
#6268=DIRECTION ( 'NONE',  ( -1.000000000000000000, 0.000000000000000000, 0.000000000000000000 ) ) ;
#6277=DIRECTION ( 'NONE',  ( 1.000000000000000000, 1.817449160981365809E-30, -1.734723475976805122E-15 ) ) ;
#6289=ORIENTED_EDGE ( 'NONE', *, *, #16719, .T. ) ;
#6297=ORIENTED_EDGE ( 'NONE', *, *, #1823, .F. ) ;
#6301=CIRCLE ( 'NONE', #2576, 1.000000000000000888 ) ;
#6310=DIRECTION ( 'NONE',  ( 0.000000000000000000, 1.000000000000000000, -2.999999999999999839E-15 ) ) ;
#6337=CARTESIAN_POINT ( 'NONE',  ( 40.31606138205700773, -31.05876147765400574, 73.55501292737010033 ) ) ;
#6338=AXIS2_PLACEMENT_3D ( 'NONE', #11343, #15183, #3336 ) ;
#6345=ADVANCED_FACE ( 'NONE', ( #2472 ), #10346, .F. ) ;
#6348=ADVANCED_FACE ( 'NONE', ( #8162 ), #2717, .T. ) ;
#6356=VECTOR ( 'NONE', #8042, 1000.000000000000000 ) ;
#6365=DIRECTION ( 'NONE',  ( -1.000000000000000000, 0.000000000000000000, 0.000000000000000000 ) ) ;
#6368=PLANE ( 'NONE',  #6912 ) ;
#6372=CYLINDRICAL_SURFACE ( 'NONE', #22099, 2.500000000000002220 ) ;
#6376=DIRECTION ( 'NONE',  ( -3.717264591378870232E-16, -2.999999999999999839E-15, -1.000000000000000000 ) ) ;
#6385=CARTESIAN_POINT ( 'NONE',  ( 36.31606138205700063, 43.19123852234596939, 66.30501292736988717 ) ) ;
#6396=AXIS2_PLACEMENT_3D ( 'NONE', #19849, #24197, #2310 ) ;
#6412=FACE_OUTER_BOUND ( 'NONE', #14357, .T. ) ;
#6428=CARTESIAN_POINT ( 'NONE',  ( 40.31606138205700773, -29.30876147765401640, 69.30501292737010033 ) ) ;
#6436=VERTEX_POINT ( 'NONE', #12796 ) ;
#6439=ORIENTED_EDGE ( 'NONE', *, *, #10957, .F. ) ;
#6440=ORIENTED_EDGE ( 'NONE', *, *, #5750, .T. ) ;
#6442=EDGE_CURVE ( 'NONE', #6126, #5370, #23213, .T. ) ;
#6443=EDGE_CURVE ( 'NONE', #14979, #22793, #15091, .T. ) ;
#6457=DIRECTION ( 'NONE',  ( 1.000000000000000000, 0.000000000000000000, 0.000000000000000000 ) ) ;
#6459=DIRECTION ( 'NONE',  ( -3.717264591378870232E-16, -3.325260651745651169E-15, -1.000000000000000000 ) ) ;
#6473=CARTESIAN_POINT ( 'NONE',  ( 43.06606138205700063, 41.44123852234599781, 74.30501292736987295 ) ) ;
#6477=EDGE_LOOP ( 'NONE', ( #9815, #4058, #16252, #9239 ) ) ;
#6479=CARTESIAN_POINT ( 'NONE',  ( 31.81606138205700418, -34.55876147765403061, 66.30501292737011454 ) ) ;
#6484=CLOSED_SHELL ( 'NONE', ( #5560, #22262, #2935, #6997, #12277, #17151, #6348, #6243, #15984, #1584, #304, #4257, #18158, #14414, #20905, #5282, #23601, #9105, #13685, #8522, #11854, #3700, #8361, #4577, #14886, #18544, #20285, #13737, #14801, #16982, #11895, #6742, #6345, #20139, #8486, #8066, #24514, #428, #6716, #24495, #9573, #17197, #646, #15537, #14220, #14340, #9553, #23026, #11476, #6089, #17433, #24524, #13589, #20845, #11320, #13557, #18022, #17114, #22463, #11061, #12151, #21097, #16486, #11432, #22068, #7044, #15812, #4196, #17617, #11970, #24964, #17144, #7322, #12867, #11058, #4690, #1857, #23231, #18628, #11626, #12259, #13559, #25140, #19548, #15021, #17473, #22393, #23868, #21353, #15988, #21148, #1413, #13129, #24649, #6557, #5013, #20812, #10847, #10278, #1872, #9730, #8343, #5717, #3575, #8432, #10988, #11628, #8875, #2318, #15248, #14754, #5494, #767, #12141, #21849, #9501, #21047, #14512, #9048, #1367, #23647, #14342, #8775, #375, #7691, #2418 ) ) ;
#6490=CARTESIAN_POINT ( 'NONE',  ( 43.06606138205700063, 41.44123852234599070, 73.55501292736987295 ) ) ;
#6494=CARTESIAN_POINT ( 'NONE',  ( 32.81606138205700773, 41.44123852234599070, 73.55501292736987295 ) ) ;
#6504=DIRECTION ( 'NONE',  ( 0.000000000000000000, 0.000000000000000000, 1.000000000000000000 ) ) ;
#6516=LINE ( 'NONE', #14625, #14976 ) ;
#6519=ORIENTED_EDGE ( 'NONE', *, *, #21800, .T. ) ;
#6530=EDGE_CURVE ( 'NONE', #12188, #21184, #14706, .T. ) ;
#6543=VECTOR ( 'NONE', #4808, 1000.000000000000000 ) ;
#6544=DIRECTION ( 'NONE',  ( 1.000000000000000000, 0.000000000000000000, 0.000000000000000000 ) ) ;
#6547=CARTESIAN_POINT ( 'NONE',  ( 31.81606138205700418, 18.19123852234599426, 73.05501292736995822 ) ) ;
#6554=VECTOR ( 'NONE', #9958, 1000.000000000000000 ) ;
#6557=ADVANCED_FACE ( 'NONE', ( #4924 ), #10860, .F. ) ;
#6560=VERTEX_POINT ( 'NONE', #19338 ) ;
#6564=CARTESIAN_POINT ( 'NONE',  ( 43.06606138205700063, 43.19123852234599070, 73.55501292736987295 ) ) ;
#6571=EDGE_CURVE ( 'NONE', #5342, #3483, #1671, .T. ) ;
#6581=EDGE_CURVE ( 'NONE', #15661, #4935, #15731, .T. ) ;
#6590=EDGE_CURVE ( 'NONE', #15938, #24485, #23318, .T. ) ;
#6600=ORIENTED_EDGE ( 'NONE', *, *, #9470, .T. ) ;
#6608=DIRECTION ( 'NONE',  ( 9.027796614315171564E-31, 1.000000000000000000, 4.694469519536151390E-16 ) ) ;
#6617=LINE ( 'NONE', #3128, #25449 ) ;
#6622=VERTEX_POINT ( 'NONE', #21401 ) ;
#6627=DIRECTION ( 'NONE',  ( 0.000000000000000000, -2.999999999999999839E-15, -1.000000000000000000 ) ) ;
#6632=ORIENTED_EDGE ( 'NONE', *, *, #20373, .F. ) ;
#6633=DIRECTION ( 'NONE',  ( 0.000000000000000000, -1.000000000000000000, 3.130104260698260371E-15 ) ) ;
#6635=ORIENTED_EDGE ( 'NONE', *, *, #7210, .T. ) ;
#6648=DIRECTION ( 'NONE',  ( 1.000000000000000000, 0.000000000000000000, 0.000000000000000000 ) ) ;
#6654=ORIENTED_EDGE ( 'NONE', *, *, #245, .F. ) ;
#6670=CARTESIAN_POINT ( 'NONE',  ( 43.81606138205700063, 35.44123852234597649, 68.80501292736990138 ) ) ;
#6671=EDGE_CURVE ( 'NONE', #11368, #22563, #11498, .T. ) ;
#6675=PLANE ( 'NONE',  #2016 ) ;
#6676=AXIS2_PLACEMENT_3D ( 'NONE', #23653, #17487, #15534 ) ;
#6687=FACE_OUTER_BOUND ( 'NONE', #3360, .T. ) ;
#6692=DIRECTION ( 'NONE',  ( 1.000000000000000000, 0.000000000000000000, 0.000000000000000000 ) ) ;
#6694=VECTOR ( 'NONE', #2597, 1000.000000000000000 ) ;
#6698=DIRECTION ( 'NONE',  ( 0.000000000000000000, -2.999999999999999839E-15, -1.000000000000000000 ) ) ;
#6702=EDGE_CURVE ( 'NONE', #13874, #13029, #20789, .T. ) ;
#6705=AXIS2_PLACEMENT_3D ( 'NONE', #25272, #17315, #11525 ) ;
#6710=CARTESIAN_POINT ( 'NONE',  ( 44.81606138205700063, 41.44123852234595518, 61.30501292736988006 ) ) ;
#6716=ADVANCED_FACE ( 'NONE', ( #19463 ), #1803, .T. ) ;
#6730=ORIENTED_EDGE ( 'NONE', *, *, #18283, .F. ) ;
#6742=ADVANCED_FACE ( 'NONE', ( #21906 ), #6070, .F. ) ;
#6745=LINE ( 'NONE', #22836, #6066 ) ;
#6750=VECTOR ( 'NONE', #10506, 1000.000000000000000 ) ;
#6755=VECTOR ( 'NONE', #25474, 1000.000000000000000 ) ;
#6757=VERTEX_POINT ( 'NONE', #2689 ) ;
#6758=ORIENTED_EDGE ( 'NONE', *, *, #16488, .T. ) ;
#6773=( GEOMETRIC_REPRESENTATION_CONTEXT ( 3 ) GLOBAL_UNCERTAINTY_ASSIGNED_CONTEXT ( ( #10308 ) ) GLOBAL_UNIT_ASSIGNED_CONTEXT ( ( #13225, #7419, #4438 ) ) REPRESENTATION_CONTEXT ( 'NONE', 'WORKASPACE' ) );
#6775=VERTEX_POINT ( 'NONE', #4270 ) ;
#6776=AXIS2_PLACEMENT_3D ( 'NONE', #20674, #1465, #22979 ) ;
#6777=ORIENTED_EDGE ( 'NONE', *, *, #14135, .F. ) ;
#6778=ORIENTED_EDGE ( 'NONE', *, *, #9594, .F. ) ;
#6781=DIRECTION ( 'NONE',  ( 1.000000000000000000, -1.301042606982604682E-30, -4.336808689942015271E-16 ) ) ;
#6783=FACE_OUTER_BOUND ( 'NONE', #6226, .T. ) ;
#6787=CARTESIAN_POINT ( 'NONE',  ( 44.81606138205700063, 28.12806996228107437, 66.30501292736992980 ) ) ;
#6794=CARTESIAN_POINT ( 'NONE',  ( 38.31606138205700063, -30.30876147765401285, 70.30501292737010033 ) ) ;
#6796=VERTEX_POINT ( 'NONE', #22153 ) ;
#6817=ORIENTED_EDGE ( 'NONE', *, *, #20893, .F. ) ;
#6823=ORIENTED_EDGE ( 'NONE', *, *, #10661, .F. ) ;
#6831=DIRECTION ( 'NONE',  ( 1.000000000000000000, -5.158740922465810421E-30, -5.611568911007197376E-44 ) ) ;
#6838=ORIENTED_EDGE ( 'NONE', *, *, #19490, .F. ) ;
#6840=CARTESIAN_POINT ( 'NONE',  ( 38.31606138205700063, 38.69123852234598360, 71.30501292737018559 ) ) ;
#6845=ORIENTED_EDGE ( 'NONE', *, *, #1540, .T. ) ;
#6846=CARTESIAN_POINT ( 'NONE',  ( 31.81606138205700418, 28.12806996228107437, 66.30501292736992980 ) ) ;
#6857=CARTESIAN_POINT ( 'NONE',  ( 33.56606138205700773, 41.44123852234595518, 61.30501292736988006 ) ) ;
#6860=DIRECTION ( 'NONE',  ( -6.056754644426120895E-31, -1.000000000000000000, -4.914813388431354887E-16 ) ) ;
#6866=DIRECTION ( 'NONE',  ( 0.000000000000000000, 1.000000000000000000, -2.999999999999999839E-15 ) ) ;
#6871=DIRECTION ( 'NONE',  ( -1.836970198721029688E-16, -2.999999999999999839E-15, -1.000000000000000000 ) ) ;
#6875=EDGE_CURVE ( 'NONE', #2367, #20177, #23670, .T. ) ;
#6890=CIRCLE ( 'NONE', #25381, 1.000000000000000888 ) ;
#6900=EDGE_CURVE ( 'NONE', #22327, #3194, #17003, .T. ) ;
#6904=LINE ( 'NONE', #19014, #9176 ) ;
#6905=EDGE_CURVE ( 'NONE', #12138, #24313, #5153, .T. ) ;
#6906=EDGE_CURVE ( 'NONE', #21318, #64, #10705, .T. ) ;
#6907=CARTESIAN_POINT ( 'NONE',  ( 35.81606138205700063, -31.05876147765399864, 75.30501292737010033 ) ) ;
#6912=AXIS2_PLACEMENT_3D ( 'NONE', #21946, #4562, #9979 ) ;
#6923=PLANE ( 'NONE',  #22732 ) ;
#6932=CARTESIAN_POINT ( 'NONE',  ( 35.81606138205700063, -31.05876147765399864, 74.30501292737010033 ) ) ;
#6938=CARTESIAN_POINT ( 'NONE',  ( 43.81606138205700063, 39.19123852234599070, 72.05501292736988717 ) ) ;
#6943=VERTEX_POINT ( 'NONE', #22539 ) ;
#6948=EDGE_CURVE ( 'NONE', #7542, #7272, #11080, .T. ) ;
#6959=DIRECTION ( 'NONE',  ( -3.469446951953614978E-15, -9.938893903907229794E-15, -1.000000000000000000 ) ) ;
#6965=EDGE_CURVE ( 'NONE', #14256, #11106, #15056, .T. ) ;
#6970=ORIENTED_EDGE ( 'NONE', *, *, #3752, .F. ) ;
#6972=VERTEX_POINT ( 'NONE', #16875 ) ;
#6985=EDGE_LOOP ( 'NONE', ( #17495, #17075, #21838, #6635 ) ) ;
#6987=CARTESIAN_POINT ( 'NONE',  ( 40.81606138205700773, -31.05876147765399864, 75.30501292737010033 ) ) ;
#6997=ADVANCED_FACE ( 'NONE', ( #5019 ), #12890, .T. ) ;
#7007=ORIENTED_EDGE ( 'NONE', *, *, #19396, .T. ) ;
#7009=CARTESIAN_POINT ( 'NONE',  ( 31.81606138205700418, 38.19123852234599070, 73.05501292736988717 ) ) ;
#7018=ORIENTED_EDGE ( 'NONE', *, *, #10135, .T. ) ;
#7027=VECTOR ( 'NONE', #19712, 1000.000000000000000 ) ;
#7034=DIRECTION ( 'NONE',  ( 0.000000000000000000, 2.999999999999998655E-15, 1.000000000000000000 ) ) ;
#7035=LINE ( 'NONE', #5115, #23021 ) ;
#7044=ADVANCED_FACE ( 'NONE', ( #1773 ), #21497, .F. ) ;
#7046=ORIENTED_EDGE ( 'NONE', *, *, #11980, .T. ) ;
#7048=DIRECTION ( 'NONE',  ( 0.000000000000000000, -1.000000000000000000, 2.999999999999999839E-15 ) ) ;
#7051=EDGE_CURVE ( 'NONE', #8061, #821, #13643, .T. ) ;
#7062=PLANE ( 'NONE',  #25168 ) ;
#7066=ORIENTED_EDGE ( 'NONE', *, *, #3670, .T. ) ;
#7067=CARTESIAN_POINT ( 'NONE',  ( 33.56606138205700773, 41.44123852234599070, 73.55501292736987295 ) ) ;
#7069=DIRECTION ( 'NONE',  ( 0.000000000000000000, 1.000000000000000000, 0.000000000000000000 ) ) ;
#7098=EDGE_LOOP ( 'NONE', ( #1987, #14459, #22120, #716 ) ) ;
#7103=AXIS2_PLACEMENT_3D ( 'NONE', #20965, #14776, #13114 ) ;
#7123=AXIS2_PLACEMENT_3D ( 'NONE', #12182, #6240, #13972 ) ;
#7125=CARTESIAN_POINT ( 'NONE',  ( 32.81606138205700773, 41.44123852234597649, 68.80501292736988717 ) ) ;
#7126=CARTESIAN_POINT ( 'NONE',  ( 31.81606138205700418, 35.38401127291550097, 61.48364296169660292 ) ) ;
#7127=AXIS2_PLACEMENT_3D ( 'NONE', #916, #13174, #20639 ) ;
#7155=VECTOR ( 'NONE', #1590, 1000.000000000000000 ) ;
#7176=VERTEX_POINT ( 'NONE', #15564 ) ;
#7181=ORIENTED_EDGE ( 'NONE', *, *, #19631, .T. ) ;
#7200=EDGE_CURVE ( 'NONE', #10392, #154, #8230, .T. ) ;
#7210=EDGE_CURVE ( 'NONE', #17867, #18276, #10290, .T. ) ;
#7221=CARTESIAN_POINT ( 'NONE',  ( 36.31606138205700063, 37.44123852234599781, 74.30501292736988717 ) ) ;
#7223=CARTESIAN_POINT ( 'NONE',  ( 38.31606138205700063, 39.69123852234598360, 70.30501292737018559 ) ) ;
#7253=DIRECTION ( 'NONE',  ( 0.000000000000000000, -1.000000000000000000, 3.325260651745651169E-15 ) ) ;
#7256=DIRECTION ( 'NONE',  ( 0.000000000000000000, -1.000000000000000000, 2.999999999999999839E-15 ) ) ;
#7272=VERTEX_POINT ( 'NONE', #22126 ) ;
#7280=VECTOR ( 'NONE', #4342, 1000.000000000000000 ) ;
#7281=ORIENTED_EDGE ( 'NONE', *, *, #22511, .T. ) ;
#7285=DIRECTION ( 'NONE',  ( 3.491481338843135327E-15, -1.000000000000000000, 2.999999999999999050E-15 ) ) ;
#7290=ORIENTED_EDGE ( 'NONE', *, *, #21527, .T. ) ;
#7301=DIRECTION ( 'NONE',  ( -1.000000000000000000, 0.000000000000000000, 0.000000000000000000 ) ) ;
#7306=ORIENTED_EDGE ( 'NONE', *, *, #1513, .T. ) ;
#7322=ADVANCED_FACE ( 'NONE', ( #16320 ), #7984, .F. ) ;
#7332=VECTOR ( 'NONE', #2898, 1000.000000000000000 ) ;
#7333=CIRCLE ( 'NONE', #10634, 0.7500000000000006661 ) ;
#7345=LINE ( 'NONE', #21004, #19287 ) ;
#7352=CYLINDRICAL_SURFACE ( 'NONE', #18085, 0.7500000000000006661 ) ;
#7354=ORIENTED_EDGE ( 'NONE', *, *, #21588, .T. ) ;
#7357=VECTOR ( 'NONE', #23174, 1000.000000000000000 ) ;
#7361=CARTESIAN_POINT ( 'NONE',  ( 43.06606138205700063, 41.44123852234599781, 75.30501292736987295 ) ) ;
#7379=FACE_BOUND ( 'NONE', #9287, .T. ) ;
#7405=EDGE_LOOP ( 'NONE', ( #2181, #3021, #13770, #10345 ) ) ;
#7406=CARTESIAN_POINT ( 'NONE',  ( 44.81606138205700063, 18.19123852234599070, 72.05501292736995822 ) ) ;
#7413=CARTESIAN_POINT ( 'NONE',  ( 31.81606138205700418, -33.00876147765401925, 70.30501292737011454 ) ) ;
#7419=( NAMED_UNIT ( * ) PLANE_ANGLE_UNIT ( ) SI_UNIT ( $, .RADIAN. ) );
#7425=DIRECTION ( 'NONE',  ( 0.000000000000000000, -1.000000000000000000, 2.999999999999999839E-15 ) ) ;
#7428=ORIENTED_EDGE ( 'NONE', *, *, #12228, .T. ) ;
#7429=EDGE_LOOP ( 'NONE', ( #8161, #10821, #15289, #16289 ) ) ;
#7433=ORIENTED_EDGE ( 'NONE', *, *, #21800, .F. ) ;
#7434=ORIENTED_EDGE ( 'NONE', *, *, #7051, .T. ) ;
#7449=CARTESIAN_POINT ( 'NONE',  ( 32.81606138205700773, 41.44123852234599070, 73.05501292736987295 ) ) ;
#7468=FACE_OUTER_BOUND ( 'NONE', #2125, .T. ) ;
#7480=ORIENTED_EDGE ( 'NONE', *, *, #24326, .T. ) ;
#7484=AXIS2_PLACEMENT_3D ( 'NONE', #20969, #1379, #13620 ) ;
#7486=DIRECTION ( 'NONE',  ( 7.386467098469070069E-45, -1.000000000000000000, 3.000000000000004177E-15 ) ) ;
#7487=AXIS2_PLACEMENT_3D ( 'NONE', #13512, #5910, #4108 ) ;
#7491=CARTESIAN_POINT ( 'NONE',  ( 31.81606138205700418, 41.44123852234596939, 66.30501292736988717 ) ) ;
#7505=AXIS2_PLACEMENT_3D ( 'NONE', #10802, #24817, #10683 ) ;
#7509=EDGE_CURVE ( 'NONE', #16850, #10286, #24299, .T. ) ;
#7525=SHAPE_REPRESENTATION ( 'Staple Magazine', ( #2000 ), #6773 ) ;
#7528=EDGE_LOOP ( 'NONE', ( #8544, #19798, #1789, #17372 ) ) ;
#7531=ORIENTED_EDGE ( 'NONE', *, *, #1692, .F. ) ;
#7536=EDGE_CURVE ( 'NONE', #11745, #4935, #5854, .T. ) ;
#7541=EDGE_LOOP ( 'NONE', ( #14798, #2150, #11777, #23009 ) ) ;
#7542=VERTEX_POINT ( 'NONE', #17354 ) ;
#7544=CARTESIAN_POINT ( 'NONE',  ( 40.81606138205700773, 41.44123852234599781, 75.30501292736988717 ) ) ;
#7557=ORIENTED_EDGE ( 'NONE', *, *, #6571, .T. ) ;
#7559=CYLINDRICAL_SURFACE ( 'NONE', #1652, 0.5000000000000004441 ) ;
#7562=CARTESIAN_POINT ( 'NONE',  ( 40.31606138205700773, 43.19123852234596939, 65.30501292736988717 ) ) ;
#7565=ORIENTED_EDGE ( 'NONE', *, *, #10147, .F. ) ;
#7566=VECTOR ( 'NONE', #14227, 1000.000000000000000 ) ;
#7578=ORIENTED_EDGE ( 'NONE', *, *, #7846, .F. ) ;
#7585=CARTESIAN_POINT ( 'NONE',  ( 31.81606138205700418, 39.19123852234599070, 72.05501292736988717 ) ) ;
#7594=CIRCLE ( 'NONE', #3888, 1.000000000000000888 ) ;
#7599=CARTESIAN_POINT ( 'NONE',  ( 35.81606138205700063, -31.05876147765399864, 75.30501292737010033 ) ) ;
#7606=CARTESIAN_POINT ( 'NONE',  ( 40.31606138205700773, -31.05876147765400574, 73.55501292737010033 ) ) ;
#7622=ORIENTED_EDGE ( 'NONE', *, *, #7210, .F. ) ;
#7658=CARTESIAN_POINT ( 'NONE',  ( 36.31606138205700063, 43.19123852234599781, 75.30501292736987295 ) ) ;
#7661=EDGE_CURVE ( 'NONE', #5882, #12862, #21096, .T. ) ;
#7663=CARTESIAN_POINT ( 'NONE',  ( 31.81606138205700418, 1.441238522345979600, 68.80501292737000085 ) ) ;
#7664=EDGE_LOOP ( 'NONE', ( #8322, #15922, #6018, #9546 ) ) ;
#7671=LINE ( 'NONE', #17208, #12065 ) ;
#7678=ORIENTED_EDGE ( 'NONE', *, *, #1840, .T. ) ;
#7680=ORIENTED_EDGE ( 'NONE', *, *, #21393, .F. ) ;
#7689=CARTESIAN_POINT ( 'NONE',  ( 40.31606138205700773, 37.44123852234599781, 74.30501292736988717 ) ) ;
#7691=ADVANCED_FACE ( 'NONE', ( #1742 ), #9641, .F. ) ;
#7707=CYLINDRICAL_SURFACE ( 'NONE', #15592, 1.550000000000002709 ) ;
#7709=CIRCLE ( 'NONE', #22100, 1.000000000000000888 ) ;
#7715=ORIENTED_EDGE ( 'NONE', *, *, #23324, .T. ) ;
#7716=EDGE_CURVE ( 'NONE', #7176, #13053, #21726, .T. ) ;
#7723=ORIENTED_EDGE ( 'NONE', *, *, #13968, .T. ) ;
#7724=DIRECTION ( 'NONE',  ( 1.000000000000000000, 0.000000000000000000, 0.000000000000000000 ) ) ;
#7730=LINE ( 'NONE', #17139, #13537 ) ;
#7736=FACE_OUTER_BOUND ( 'NONE', #7405, .T. ) ;
#7740=EDGE_CURVE ( 'NONE', #22901, #18207, #4081, .T. ) ;
#7749=DIRECTION ( 'NONE',  ( -1.000000000000000000, 0.000000000000000000, 0.000000000000000000 ) ) ;
#7753=CARTESIAN_POINT ( 'NONE',  ( 40.31606138205700773, -29.30876147765400219, 74.30501292737010033 ) ) ;
#7754=FACE_OUTER_BOUND ( 'NONE', #13827, .T. ) ;
#7761=VECTOR ( 'NONE', #8726, 1000.000000000000000 ) ;
#7771=VECTOR ( 'NONE', #23229, 1000.000000000000000 ) ;
#7776=ORIENTED_EDGE ( 'NONE', *, *, #10837, .T. ) ;
#7780=DIRECTION ( 'NONE',  ( 0.000000000000000000, 2.999999999999999839E-15, 1.000000000000000000 ) ) ;
#7792=ORIENTED_EDGE ( 'NONE', *, *, #15127, .T. ) ;
#7796=LINE ( 'NONE', #15643, #3170 ) ;
#7800=VECTOR ( 'NONE', #14954, 1000.000000000000000 ) ;
#7806=AXIS2_PLACEMENT_3D ( 'NONE', #1389, #16986, #17236 ) ;
#7811=CARTESIAN_POINT ( 'NONE',  ( 36.31606138205700063, -29.30876147765401640, 69.30501292737010033 ) ) ;
#7812=AXIS2_PLACEMENT_3D ( 'NONE', #4729, #22371, #12843 ) ;
#7818=DIRECTION ( 'NONE',  ( 0.000000000000000000, 1.000000000000000000, 0.000000000000000000 ) ) ;
#7827=ORIENTED_EDGE ( 'NONE', *, *, #13984, .T. ) ;
#7828=DIRECTION ( 'NONE',  ( -1.000000000000000000, 0.000000000000000000, 0.000000000000000000 ) ) ;
#7846=EDGE_CURVE ( 'NONE', #9967, #5642, #4928, .T. ) ;
#7850=DIRECTION ( 'NONE',  ( -4.789116818843729608E-32, 1.000000000000000000, -3.130104260698260371E-15 ) ) ;
#7852=VECTOR ( 'NONE', #12097, 1000.000000000000000 ) ;
#7859=ORIENTED_EDGE ( 'NONE', *, *, #23995, .T. ) ;
#7860=FILL_AREA_STYLE_COLOUR ( '', #1192 ) ;
#7862=PLANE ( 'NONE',  #22373 ) ;
#7870=FACE_OUTER_BOUND ( 'NONE', #8511, .T. ) ;
#7871=CARTESIAN_POINT ( 'NONE',  ( 44.81606138205700063, 35.44123852234597649, 68.30501292736990138 ) ) ;
#7882=EDGE_LOOP ( 'NONE', ( #7792, #5807, #2471, #13753 ) ) ;
#7883=DIRECTION ( 'NONE',  ( -7.570943305532639295E-31, -1.000000000000000000, -4.914813388431354887E-16 ) ) ;
#7890=CIRCLE ( 'NONE', #472, 2.500000000000002220 ) ;
#7904=VERTEX_POINT ( 'NONE', #21657 ) ;
#7906=EDGE_LOOP ( 'NONE', ( #19429, #11144, #23693, #6823 ) ) ;
#7908=LINE ( 'NONE', #19364, #16997 ) ;
#7910=ORIENTED_EDGE ( 'NONE', *, *, #16177, .T. ) ;
#7913=DIRECTION ( 'NONE',  ( 0.000000000000000000, -1.000000000000000000, 2.999999999999999839E-15 ) ) ;
#7917=VECTOR ( 'NONE', #10864, 1000.000000000000000 ) ;
#7925=CARTESIAN_POINT ( 'NONE',  ( 43.81606138205700063, 41.44123852234598360, 71.05501292736988717 ) ) ;
#7929=PRESENTATION_STYLE_ASSIGNMENT (( #13844 ) ) ;
#7930=CARTESIAN_POINT ( 'NONE',  ( 38.31606138205712853, 42.19123852234595518, 61.30501292736988006 ) ) ;
#7933=VECTOR ( 'NONE', #5411, 1000.000000000000000 ) ;
#7949=CARTESIAN_POINT ( 'NONE',  ( 43.06606138205700063, 41.44123852234599781, 75.30501292736987295 ) ) ;
#7953=LINE ( 'NONE', #21724, #21044 ) ;
#7956=VECTOR ( 'NONE', #7961, 1000.000000000000000 ) ;
#7959=ORIENTED_EDGE ( 'NONE', *, *, #7740, .T. ) ;
#7961=DIRECTION ( 'NONE',  ( 3.491481338843135327E-15, 1.000000000000000000, -2.999999999999999839E-15 ) ) ;
#7966=CARTESIAN_POINT ( 'NONE',  ( 44.81606138205700063, -34.55876147765400930, 73.30501292737011454 ) ) ;
#7971=ORIENTED_EDGE ( 'NONE', *, *, #5256, .T. ) ;
#7980=FACE_OUTER_BOUND ( 'NONE', #5292, .T. ) ;
#7984=PLANE ( 'NONE',  #21509 ) ;
#7985=VECTOR ( 'NONE', #19720, 1000.000000000000000 ) ;
#7991=DIRECTION ( 'NONE',  ( 0.000000000000000000, -2.999999999999999839E-15, -1.000000000000000000 ) ) ;
#8003=ORIENTED_EDGE ( 'NONE', *, *, #21070, .F. ) ;
#8041=ORIENTED_EDGE ( 'NONE', *, *, #11635, .T. ) ;
#8042=DIRECTION ( 'NONE',  ( -1.000000000000000000, 0.000000000000000000, 0.000000000000000000 ) ) ;
#8050=CARTESIAN_POINT ( 'NONE',  ( 35.81606138205700063, -24.05876147765400219, 74.30501292737008612 ) ) ;
#8054=CARTESIAN_POINT ( 'NONE',  ( 44.81606138205700063, -34.55876147765400930, 73.30501292737011454 ) ) ;
#8061=VERTEX_POINT ( 'NONE', #4146 ) ;
#8063=VERTEX_POINT ( 'NONE', #25114 ) ;
#8064=ORIENTED_EDGE ( 'NONE', *, *, #1119, .T. ) ;
#8066=ADVANCED_FACE ( 'NONE', ( #9698, #14191 ), #24081, .F. ) ;
#8073=LINE ( 'NONE', #6135, #1264 ) ;
#8081=ORIENTED_EDGE ( 'NONE', *, *, #9594, .T. ) ;
#8083=DIRECTION ( 'NONE',  ( 0.000000000000000000, 1.000000000000000000, -2.999999999999998655E-15 ) ) ;
#8085=EDGE_CURVE ( 'NONE', #21126, #17867, #8649, .T. ) ;
#8093=EDGE_LOOP ( 'NONE', ( #15997, #16811, #6632, #24378 ) ) ;
#8104=DIRECTION ( 'NONE',  ( 1.000000000000000000, -1.301042606982604682E-30, -4.336808689942015271E-16 ) ) ;
#8107=AXIS2_PLACEMENT_3D ( 'NONE', #826, #2884, #18749 ) ;
#8122=LINE ( 'NONE', #4636, #7027 ) ;
#8143=AXIS2_PLACEMENT_3D ( 'NONE', #1969, #13342, #5472 ) ;
#8144=VECTOR ( 'NONE', #20558, 1000.000000000000114 ) ;
#8161=ORIENTED_EDGE ( 'NONE', *, *, #14678, .F. ) ;
#8162=FACE_OUTER_BOUND ( 'NONE', #5613, .T. ) ;
#8167=FACE_OUTER_BOUND ( 'NONE', #3413, .T. ) ;
#8170=CARTESIAN_POINT ( 'NONE',  ( 43.06606138205700063, 42.19123852234599781, 74.30501292736987295 ) ) ;
#8172=ORIENTED_EDGE ( 'NONE', *, *, #3284, .T. ) ;
#8184=VECTOR ( 'NONE', #16023, 1000.000000000000000 ) ;
#8193=ORIENTED_EDGE ( 'NONE', *, *, #12417, .T. ) ;
#8195=PLANE ( 'NONE',  #18147 ) ;
#8196=FACE_BOUND ( 'NONE', #17765, .T. ) ;
#8213=CARTESIAN_POINT ( 'NONE',  ( 36.31606138205700063, 38.69123852234599070, 73.55501292736988717 ) ) ;
#8215=LINE ( 'NONE', #14264, #16013 ) ;
#8225=EDGE_LOOP ( 'NONE', ( #20569, #20634, #22497, #2, #10807 ) ) ;
#8230=LINE ( 'NONE', #14404, #1744 ) ;
#8233=CARTESIAN_POINT ( 'NONE',  ( 38.31606138205700063, 42.51966564709218233, 71.30501292737018559 ) ) ;
#8243=VERTEX_POINT ( 'NONE', #14309 ) ;
#8244=VECTOR ( 'NONE', #25240, 1000.000000000000000 ) ;
#8256=DIRECTION ( 'NONE',  ( 0.000000000000000000, -6.938893903907222067E-15, 1.000000000000000000 ) ) ;
#8269=DIRECTION ( 'NONE',  ( 1.000000000000000000, -6.938893903907222067E-15, 0.000000000000000000 ) ) ;
#8280=ORIENTED_EDGE ( 'NONE', *, *, #8581, .T. ) ;
#8285=CARTESIAN_POINT ( 'NONE',  ( 31.81606138205700418, 35.44123852234597649, 68.30501292736990138 ) ) ;
#8286=AXIS2_PLACEMENT_3D ( 'NONE', #1873, #13487, #9638 ) ;
#8298=ORIENTED_EDGE ( 'NONE', *, *, #22816, .T. ) ;
#8300=EDGE_CURVE ( 'NONE', #10990, #6757, #10828, .T. ) ;
#8301=CARTESIAN_POINT ( 'NONE',  ( 38.31606138205700063, 39.69123852234599070, 72.30501292737018559 ) ) ;
#8312=DIRECTION ( 'NONE',  ( -3.083952846180990083E-15, 1.000000000000000000, -2.999999999999998655E-15 ) ) ;
#8315=LINE ( 'NONE', #17860, #22257 ) ;
#8317=VERTEX_POINT ( 'NONE', #8776 ) ;
#8318=DIRECTION ( 'NONE',  ( 0.000000000000000000, 1.000000000000000000, -2.999999999999998655E-15 ) ) ;
#8322=ORIENTED_EDGE ( 'NONE', *, *, #17911, .F. ) ;
#8326=FACE_OUTER_BOUND ( 'NONE', #24275, .T. ) ;
#8332=DIRECTION ( 'NONE',  ( 0.000000000000000000, 2.775557561562888984E-15, 1.000000000000000000 ) ) ;
#8340=DIRECTION ( 'NONE',  ( -1.000000000000000000, 3.491481338843135327E-15, -1.047444401652940473E-29 ) ) ;
#8343=ADVANCED_FACE ( 'NONE', ( #13273 ), #9295, .T. ) ;
#8345=AXIS2_PLACEMENT_3D ( 'NONE', #23275, #9649, #3450 ) ;
#8347=CARTESIAN_POINT ( 'NONE',  ( 40.31606138205700773, 37.94123852234599070, 73.55501292736988717 ) ) ;
#8361=ADVANCED_FACE ( 'NONE', ( #13017, #4894 ), #9790, .T. ) ;
#8364=AXIS2_PLACEMENT_3D ( 'NONE', #13466, #23494, #22992 ) ;
#8365=DIRECTION ( 'NONE',  ( -4.336808689942015271E-16, 4.914813388431354887E-16, -1.000000000000000000 ) ) ;
#8370=CIRCLE ( 'NONE', #11246, 0.5000000000000004441 ) ;
#8371=CARTESIAN_POINT ( 'NONE',  ( 35.31606138205687273, 42.19123852234599781, 75.30501292736987295 ) ) ;
#8376=CARTESIAN_POINT ( 'NONE',  ( 40.31606138205700773, -30.30876147765400574, 73.55501292737010033 ) ) ;
#8379=ORIENTED_EDGE ( 'NONE', *, *, #11831, .T. ) ;
#8387=FACE_OUTER_BOUND ( 'NONE', #23235, .T. ) ;
#8398=MANIFOLD_SOLID_BREP ( 'NONE', #6484 ) ;
#8403=VECTOR ( 'NONE', #21245, 1000.000000000000000 ) ;
#8410=( GEOMETRIC_REPRESENTATION_CONTEXT ( 3 ) GLOBAL_UNCERTAINTY_ASSIGNED_CONTEXT ( ( #18793 ) ) GLOBAL_UNIT_ASSIGNED_CONTEXT ( ( #11924, #1975, #46 ) ) REPRESENTATION_CONTEXT ( 'NONE', 'WORKASPACE' ) );
#8415=CARTESIAN_POINT ( 'NONE',  ( 43.81606138205700063, 41.44123852234596939, 66.30501292736988717 ) ) ;
#8425=CARTESIAN_POINT ( 'NONE',  ( 44.81606138205700063, -38.55876147765401640, 71.30501292737012875 ) ) ;
#8432=ADVANCED_FACE ( 'NONE', ( #17258, #3714, #1521, #1779 ), #5919, .F. ) ;
#8442=VERTEX_POINT ( 'NONE', #9671 ) ;
#8444=CYLINDRICAL_SURFACE ( 'NONE', #19728, 0.5000000000000004441 ) ;
#8451=ORIENTED_EDGE ( 'NONE', *, *, #19820, .T. ) ;
#8459=DIRECTION ( 'NONE',  ( 0.000000000000000000, 0.000000000000000000, 1.000000000000000000 ) ) ;
#8462=ORIENTED_EDGE ( 'NONE', *, *, #24940, .F. ) ;
#8473=EDGE_LOOP ( 'NONE', ( #3101, #23674, #6838, #17485 ) ) ;
#8474=ORIENTED_EDGE ( 'NONE', *, *, #1196, .T. ) ;
#8481=EDGE_LOOP ( 'NONE', ( #1558, #21600, #10008, #25016 ) ) ;
#8482=ORIENTED_EDGE ( 'NONE', *, *, #16965, .T. ) ;
#8486=ADVANCED_FACE ( 'NONE', ( #7468 ), #21756, .T. ) ;
#8491=DIRECTION ( 'NONE',  ( -1.836970198721029688E-16, -2.999999999999999839E-15, -1.000000000000000000 ) ) ;
#8492=FACE_OUTER_BOUND ( 'NONE', #15008, .T. ) ;
#8501=CARTESIAN_POINT ( 'NONE',  ( 41.81606138205687273, 43.19123852234595518, 61.30501292736988006 ) ) ;
#8511=EDGE_LOOP ( 'NONE', ( #2258, #12573, #7715, #5724 ) ) ;
#8522=ADVANCED_FACE ( 'NONE', ( #478 ), #4620, .F. ) ;
#8526=EDGE_CURVE ( 'NONE', #22825, #11106, #10294, .T. ) ;
#8529=ORIENTED_EDGE ( 'NONE', *, *, #1582, .T. ) ;
#8537=ORIENTED_EDGE ( 'NONE', *, *, #16586, .T. ) ;
#8539=ORIENTED_EDGE ( 'NONE', *, *, #11311, .T. ) ;
#8544=ORIENTED_EDGE ( 'NONE', *, *, #4197, .F. ) ;
#8554=VECTOR ( 'NONE', #13837, 1000.000000000000000 ) ;
#8563=DIRECTION ( 'NONE',  ( -1.000000000000000000, 5.510910596163088391E-31, 1.836970198721029688E-16 ) ) ;
#8581=EDGE_CURVE ( 'NONE', #22825, #8063, #10279, .T. ) ;
#8583=ORIENTED_EDGE ( 'NONE', *, *, #5103, .F. ) ;
#8592=DIRECTION ( 'NONE',  ( -3.083952846180990083E-15, -1.000000000000000000, 2.999999999999999839E-15 ) ) ;
#8602=CARTESIAN_POINT ( 'NONE',  ( 40.31606138205700773, 42.19123852234599781, 75.30501292736987295 ) ) ;
#8609=DIRECTION ( 'NONE',  ( 0.000000000000000000, 1.000000000000000000, 0.000000000000000000 ) ) ;
#8620=EDGE_CURVE ( 'NONE', #1727, #11848, #16323, .T. ) ;
#8625=FACE_OUTER_BOUND ( 'NONE', #7528, .T. ) ;
#8628=ORIENTED_EDGE ( 'NONE', *, *, #10858, .T. ) ;
#8629=DIRECTION ( 'NONE',  ( -1.000000000000000000, 0.000000000000000000, 0.000000000000000000 ) ) ;
#8630=CARTESIAN_POINT ( 'NONE',  ( 33.56606138205700773, 42.19123852234599070, 73.55501292736987295 ) ) ;
#8649=LINE ( 'NONE', #23956, #13586 ) ;
#8650=CIRCLE ( 'NONE', #18102, 1.750000000000001554 ) ;
#8659=FACE_OUTER_BOUND ( 'NONE', #6477, .T. ) ;
#8667=DIRECTION ( 'NONE',  ( 0.000000000000000000, 1.000000000000000000, -2.999999999999999839E-15 ) ) ;
#8678=DIRECTION ( 'NONE',  ( 1.836970198721029688E-16, 2.999999999999999839E-15, 1.000000000000000000 ) ) ;
#8681=DIRECTION ( 'NONE',  ( -8.673617379884039170E-17, 1.163336342344340343E-15, -1.000000000000000000 ) ) ;
#8693=AXIS2_PLACEMENT_3D ( 'NONE', #13995, #17991, #5621 ) ;
#8694=DIRECTION ( 'NONE',  ( 0.000000000000000000, 3.469446951953611033E-15, 1.000000000000000000 ) ) ;
#8710=FACE_BOUND ( 'NONE', #29, .T. ) ;
#8716=CYLINDRICAL_SURFACE ( 'NONE', #8107, 1.550000000000002709 ) ;
#8718=EDGE_LOOP ( 'NONE', ( #6107, #3604, #11189, #16220, #9507, #14271 ) ) ;
#8720=ORIENTED_EDGE ( 'NONE', *, *, #10957, .T. ) ;
#8724=LINE ( 'NONE', #24406, #24172 ) ;
#8725=CARTESIAN_POINT ( 'NONE',  ( 36.31606138205700063, -29.30876147765401640, 69.30501292737010033 ) ) ;
#8726=DIRECTION ( 'NONE',  ( 1.000000000000000000, 0.000000000000000000, 0.000000000000000000 ) ) ;
#8731=ORIENTED_EDGE ( 'NONE', *, *, #24497, .F. ) ;
#8733=CIRCLE ( 'NONE', #13670, 1.000000000000000888 ) ;
#8738=ORIENTED_EDGE ( 'NONE', *, *, #18084, .F. ) ;
#8752=CIRCLE ( 'NONE', #15321, 1.550000000000002709 ) ;
#8760=EDGE_LOOP ( 'NONE', ( #1592, #24501, #22780, #23402 ) ) ;
#8775=ADVANCED_FACE ( 'NONE', ( #3053 ), #10929, .F. ) ;
#8776=CARTESIAN_POINT ( 'NONE',  ( 34.81606138205687273, 42.19123852234595518, 61.30501292736988006 ) ) ;
#8780=CIRCLE ( 'NONE', #23152, 1.000000000000000888 ) ;
#8789=ORIENTED_EDGE ( 'NONE', *, *, #3484, .T. ) ;
#8792=ORIENTED_EDGE ( 'NONE', *, *, #14135, .T. ) ;
#8796=VERTEX_POINT ( 'NONE', #24871 ) ;
#8823=FACE_OUTER_BOUND ( 'NONE', #1397, .T. ) ;
#8848=VERTEX_POINT ( 'NONE', #5317 ) ;
#8849=VERTEX_POINT ( 'NONE', #8930 ) ;
#8875=ADVANCED_FACE ( 'NONE', ( #22574, #24743, #7379, #24610 ), #18838, .T. ) ;
#8884=DIRECTION ( 'NONE',  ( -1.000000000000000000, -6.938893903907222067E-15, 0.000000000000000000 ) ) ;
#8897=CARTESIAN_POINT ( 'NONE',  ( 44.81606138205700063, -24.55876147765400574, 72.80501292737008612 ) ) ;
#8906=ORIENTED_EDGE ( 'NONE', *, *, #17941, .T. ) ;
#8917=ORIENTED_EDGE ( 'NONE', *, *, #17637, .F. ) ;
#8924=CARTESIAN_POINT ( 'NONE',  ( 38.31606138205700063, 38.69123852234598360, 71.30501292737018559 ) ) ;
#8925=PLANE ( 'NONE',  #3830 ) ;
#8930=CARTESIAN_POINT ( 'NONE',  ( 36.31606138205700063, 42.19123852234596939, 65.30501292736988717 ) ) ;
#8933=LINE ( 'NONE', #5066, #5921 ) ;
#8984=VECTOR ( 'NONE', #1352, 1000.000000000000000 ) ;
#8987=ORIENTED_EDGE ( 'NONE', *, *, #13879, .F. ) ;
#8993=DIRECTION ( 'NONE',  ( -1.000000000000000000, 5.510910596163088391E-31, 1.836970198721029688E-16 ) ) ;
#9001=DIRECTION ( 'NONE',  ( 0.000000000000000000, -3.965082230804126670E-15, -1.000000000000000000 ) ) ;
#9002=EDGE_CURVE ( 'NONE', #9093, #6757, #6077, .T. ) ;
#9009=VECTOR ( 'NONE', #18306, 1000.000000000000000 ) ;
#9012=DIRECTION ( 'NONE',  ( 1.000000000000000000, 0.000000000000000000, 0.000000000000000000 ) ) ;
#9013=CARTESIAN_POINT ( 'NONE',  ( 43.81606138205700063, 41.44123852234599070, 73.55501292736987295 ) ) ;
#9021=LINE ( 'NONE', #10818, #18964 ) ;
#9047=DIRECTION ( 'NONE',  ( 1.000000000000000000, 0.000000000000000000, 0.000000000000000000 ) ) ;
#9048=ADVANCED_FACE ( 'NONE', ( #15351 ), #23323, .F. ) ;
#9060=CIRCLE ( 'NONE', #9460, 1.549999999999995826 ) ;
#9070=CARTESIAN_POINT ( 'NONE',  ( 31.81606138205700418, 41.44123852234599781, 75.30501292736988717 ) ) ;
#9071=DIRECTION ( 'NONE',  ( 1.000000000000000000, 0.000000000000000000, 0.000000000000000000 ) ) ;
#9086=ORIENTED_EDGE ( 'NONE', *, *, #20456, .F. ) ;
#9088=CARTESIAN_POINT ( 'NONE',  ( 31.81606138205700418, 41.44123852234599070, 73.55501292736987295 ) ) ;
#9090=AXIS2_PLACEMENT_3D ( 'NONE', #15553, #19417, #25330 ) ;
#9093=VERTEX_POINT ( 'NONE', #4276 ) ;
#9101=LINE ( 'NONE', #16942, #17996 ) ;
#9105=ADVANCED_FACE ( 'NONE', ( #763 ), #16355, .F. ) ;
#9106=ORIENTED_EDGE ( 'NONE', *, *, #18939, .F. ) ;
#9107=DIRECTION ( 'NONE',  ( -1.000000000000000000, 1.115179377413661005E-30, 3.717264591378870232E-16 ) ) ;
#9108=VECTOR ( 'NONE', #6633, 1000.000000000000000 ) ;
#9127=CARTESIAN_POINT ( 'NONE',  ( 44.81606138205700063, 41.44123852234599781, 74.30501292736987295 ) ) ;
#9142=AXIS2_PLACEMENT_3D ( 'NONE', #18394, #24296, #8609 ) ;
#9144=ORIENTED_EDGE ( 'NONE', *, *, #5659, .F. ) ;
#9148=ORIENTED_EDGE ( 'NONE', *, *, #9177, .T. ) ;
#9156=CARTESIAN_POINT ( 'NONE',  ( 36.31606138205700063, 41.44123852234599781, 74.30501292736987295 ) ) ;
#9160=ORIENTED_EDGE ( 'NONE', *, *, #11446, .F. ) ;
#9166=AXIS2_PLACEMENT_3D ( 'NONE', #18941, #10954, #5159 ) ;
#9176=VECTOR ( 'NONE', #6648, 1000.000000000000000 ) ;
#9177=EDGE_CURVE ( 'NONE', #10587, #24927, #19856, .T. ) ;
#9188=DIRECTION ( 'NONE',  ( 0.000000000000000000, 6.938893903907222067E-15, -1.000000000000000000 ) ) ;
#9195=DIRECTION ( 'NONE',  ( -1.000000000000000000, 1.040834085586084551E-30, 3.469446951953615175E-16 ) ) ;
#9202=FACE_OUTER_BOUND ( 'NONE', #24651, .T. ) ;
#9210=CIRCLE ( 'NONE', #23580, 1.000000000000000888 ) ;
#9219=CIRCLE ( 'NONE', #3842, 0.7500000000000006661 ) ;
#9220=DIRECTION ( 'NONE',  ( 0.000000000000000000, -4.625929269271481378E-15, -1.000000000000000000 ) ) ;
#9226=PLANE ( 'NONE',  #16141 ) ;
#9239=ORIENTED_EDGE ( 'NONE', *, *, #1823, .T. ) ;
#9245=VECTOR ( 'NONE', #9668, 1000.000000000000000 ) ;
#9249=CARTESIAN_POINT ( 'NONE',  ( 38.31606138205700063, -29.30876147765399864, 75.30501292736995822 ) ) ;
#9260=LINE ( 'NONE', #3684, #23902 ) ;
#9269=PLANE ( 'NONE',  #7505 ) ;
#9282=EDGE_CURVE ( 'NONE', #154, #20176, #19069, .T. ) ;
#9284=LINE ( 'NONE', #24349, #3364 ) ;
#9286=CARTESIAN_POINT ( 'NONE',  ( 0.000000000000000000, 0.000000000000000000, 0.000000000000000000 ) ) ;
#9287=EDGE_LOOP ( 'NONE', ( #10187, #20379, #6777, #14454, #9160 ) ) ;
#9293=EDGE_CURVE ( 'NONE', #2891, #16994, #22787, .T. ) ;
#9295=PLANE ( 'NONE',  #6144 ) ;
#9297=DIRECTION ( 'NONE',  ( 0.000000000000000000, -0.8213699656732942334, 0.5703958094953462954 ) ) ;
#9298=CARTESIAN_POINT ( 'NONE',  ( 44.81606138205700063, 39.19123852234599070, 72.05501292736988717 ) ) ;
#9300=LINE ( 'NONE', #25089, #1381 ) ;
#9303=ORIENTED_EDGE ( 'NONE', *, *, #20835, .F. ) ;
#9307=ORIENTED_EDGE ( 'NONE', *, *, #2320, .T. ) ;
#9311=PRODUCT ( 'Staple Magazine', 'Staple Magazine', '', ( #18979 ) ) ;
#9316=LINE ( 'NONE', #19210, #5258 ) ;
#9324=DIRECTION ( 'NONE',  ( -9.027796614315171564E-31, -1.000000000000000000, -3.938893903907230117E-15 ) ) ;
#9333=DIRECTION ( 'NONE',  ( -3.717264591378870232E-16, -2.999999999999999839E-15, -1.000000000000000000 ) ) ;
#9337=ORIENTED_EDGE ( 'NONE', *, *, #409, .F. ) ;
#9339=ORIENTED_EDGE ( 'NONE', *, *, #18084, .T. ) ;
#9344=ORIENTED_EDGE ( 'NONE', *, *, #409, .T. ) ;
#9350=DIRECTION ( 'NONE',  ( -3.373073425510455500E-16, -2.999999999999999839E-15, -1.000000000000000000 ) ) ;
#9356=CIRCLE ( 'NONE', #15087, 1.000000000000000888 ) ;
#9366=VERTEX_POINT ( 'NONE', #24846 ) ;
#9370=ORIENTED_EDGE ( 'NONE', *, *, #16976, .F. ) ;
#9374=AXIS2_PLACEMENT_3D ( 'NONE', #19393, #25426, #1864 ) ;
#9376=ORIENTED_EDGE ( 'NONE', *, *, #8526, .T. ) ;
#9377=VERTEX_POINT ( 'NONE', #7221 ) ;
#9381=CARTESIAN_POINT ( 'NONE',  ( 35.31606138205687273, 43.19123852234595518, 61.30501292736988006 ) ) ;
#9386=VECTOR ( 'NONE', #20355, 1000.000000000000000 ) ;
#9397=EDGE_LOOP ( 'NONE', ( #9086, #2010, #6970, #11908 ) ) ;
#9408=ORIENTED_EDGE ( 'NONE', *, *, #19959, .T. ) ;
#9418=DIRECTION ( 'NONE',  ( -1.000000000000000000, 5.352861011585579840E-16, -1.605858303475673768E-30 ) ) ;
#9424=LINE ( 'NONE', #17397, #15191 ) ;
#9429=VERTEX_POINT ( 'NONE', #25479 ) ;
#9434=CARTESIAN_POINT ( 'NONE',  ( 36.31606138205700063, 37.94123852234599070, 73.55501292736988717 ) ) ;
#9439=CARTESIAN_POINT ( 'NONE',  ( 40.31606138205700773, -29.30876147765401640, 69.30501292737010033 ) ) ;
#9440=DIRECTION ( 'NONE',  ( -1.000000000000000000, 5.510910596163088391E-31, 1.836970198721029688E-16 ) ) ;
#9457=LINE ( 'NONE', #17306, #2809 ) ;
#9460=AXIS2_PLACEMENT_3D ( 'NONE', #4128, #5804, #21514 ) ;
#9464=ORIENTED_EDGE ( 'NONE', *, *, #1692, .T. ) ;
#9470=EDGE_CURVE ( 'NONE', #21084, #11800, #11598, .T. ) ;
#9472=DIRECTION ( 'NONE',  ( 1.000000000000000000, -8.673617379884029556E-16, 2.602085213965208662E-30 ) ) ;
#9476=AXIS2_PLACEMENT_3D ( 'NONE', #9801, #13364, #21640 ) ;
#9478=CARTESIAN_POINT ( 'NONE',  ( 43.81606138205700063, -24.55876147765401285, 70.30501292737008612 ) ) ;
#9485=DIRECTION ( 'NONE',  ( 0.000000000000000000, -1.000000000000000000, 2.999999999999999839E-15 ) ) ;
#9492=ORIENTED_EDGE ( 'NONE', *, *, #16777, .F. ) ;
#9496=ORIENTED_EDGE ( 'NONE', *, *, #7536, .F. ) ;
#9501=ADVANCED_FACE ( 'NONE', ( #19695 ), #13402, .F. ) ;
#9506=DIRECTION ( 'NONE',  ( 1.000000000000000000, -5.204170427930415223E-30, -1.734723475976805122E-15 ) ) ;
#9507=ORIENTED_EDGE ( 'NONE', *, *, #5256, .F. ) ;
#9511=DIRECTION ( 'NONE',  ( 0.000000000000000000, 2.999999999999999839E-15, 1.000000000000000000 ) ) ;
#9514=CIRCLE ( 'NONE', #18560, 1.550000000000002709 ) ;
#9531=CARTESIAN_POINT ( 'NONE',  ( 40.81606138205700773, -24.05876147765399864, 75.30501292737008612 ) ) ;
#9535=CARTESIAN_POINT ( 'NONE',  ( 31.81606138205700418, 41.44123852234599070, 73.55501292736987295 ) ) ;
#9537=VERTEX_POINT ( 'NONE', #23293 ) ;
#9546=ORIENTED_EDGE ( 'NONE', *, *, #5165, .T. ) ;
#9553=ADVANCED_FACE ( 'NONE', ( #11349 ), #9919, .F. ) ;
#9558=FACE_OUTER_BOUND ( 'NONE', #16636, .T. ) ;
#9573=ADVANCED_FACE ( 'NONE', ( #5658 ), #17260, .T. ) ;
#9575=EDGE_LOOP ( 'NONE', ( #9624, #15399, #13572, #23155 ) ) ;
#9576=LINE ( 'NONE', #5443, #20886 ) ;
#9583=CIRCLE ( 'NONE', #18220, 0.7500000000000006661 ) ;
#9594=EDGE_CURVE ( 'NONE', #25151, #5023, #17809, .T. ) ;
#9606=AXIS2_PLACEMENT_3D ( 'NONE', #24151, #2394, #18134 ) ;
#9610=ORIENTED_EDGE ( 'NONE', *, *, #20835, .T. ) ;
#9615=CARTESIAN_POINT ( 'NONE',  ( 40.31606138205700773, 42.19123852234596939, 66.30501292736988717 ) ) ;
#9616=DIRECTION ( 'NONE',  ( 1.000000000000000000, 0.000000000000000000, 0.000000000000000000 ) ) ;
#9622=CARTESIAN_POINT ( 'NONE',  ( 31.81606138205700418, 32.99511671078946762, 63.14259751872857152 ) ) ;
#9624=ORIENTED_EDGE ( 'NONE', *, *, #20700, .T. ) ;
#9638=DIRECTION ( 'NONE',  ( 0.000000000000000000, -1.000000000000000000, 3.469446951953617344E-15 ) ) ;
#9641=CYLINDRICAL_SURFACE ( 'NONE', #15722, 2.500000000000002220 ) ;
#9649=DIRECTION ( 'NONE',  ( -1.000000000000000000, 1.678764654171101651E-30, 5.595882180570339263E-16 ) ) ;
#9661=ORIENTED_EDGE ( 'NONE', *, *, #14374, .T. ) ;
#9668=DIRECTION ( 'NONE',  ( 0.000000000000000000, 1.000000000000000000, -2.913263826201159484E-15 ) ) ;
#9671=CARTESIAN_POINT ( 'NONE',  ( 34.56606138205700773, 42.19123852234599781, 75.30501292736987295 ) ) ;
#9676=CARTESIAN_POINT ( 'NONE',  ( 31.81606138205700418, 38.19123852234598360, 71.05501292736988717 ) ) ;
#9677=DIRECTION ( 'NONE',  ( 1.734723475976805122E-15, 2.999999999999999839E-15, 1.000000000000000000 ) ) ;
#9684=ORIENTED_EDGE ( 'NONE', *, *, #3341, .F. ) ;
#9685=ORIENTED_EDGE ( 'NONE', *, *, #1761, .F. ) ;
#9698=FACE_BOUND ( 'NONE', #5093, .T. ) ;
#9702=CARTESIAN_POINT ( 'NONE',  ( 31.81606138205700418, 38.19123852234599070, 72.05501292736988717 ) ) ;
#9718=ORIENTED_EDGE ( 'NONE', *, *, #6442, .T. ) ;
#9720=CARTESIAN_POINT ( 'NONE',  ( 33.56606138205700773, 41.44123852234599070, 73.55501292736987295 ) ) ;
#9728=ORIENTED_EDGE ( 'NONE', *, *, #22773, .T. ) ;
#9730=ADVANCED_FACE ( 'NONE', ( #8492 ), #23803, .T. ) ;
#9731=DIRECTION ( 'NONE',  ( -3.224213076541129652E-32, -1.000000000000000000, 2.913263826201159484E-15 ) ) ;
#9744=ORIENTED_EDGE ( 'NONE', *, *, #21754, .F. ) ;
#9746=PLANE ( 'NONE',  #16910 ) ;
#9748=ORIENTED_EDGE ( 'NONE', *, *, #18945, .T. ) ;
#9756=DIRECTION ( 'NONE',  ( 0.000000000000000000, 0.000000000000000000, -1.000000000000000000 ) ) ;
#9757=EDGE_LOOP ( 'NONE', ( #9337, #17145, #24384, #18618 ) ) ;
#9772=AXIS2_PLACEMENT_3D ( 'NONE', #9702, #23076, #17552 ) ;
#9790=PLANE ( 'NONE',  #4899 ) ;
#9794=DIRECTION ( 'NONE',  ( -4.836319614811699678E-32, 1.000000000000000000, -3.130104260698260371E-15 ) ) ;
#9795=CARTESIAN_POINT ( 'NONE',  ( 36.31606138205700063, 37.94123852234599781, 74.30501292736988717 ) ) ;
#9796=CARTESIAN_POINT ( 'NONE',  ( 44.81606138205700063, -22.55876147765401996, 68.80501292737008612 ) ) ;
#9801=CARTESIAN_POINT ( 'NONE',  ( 31.81606138205700418, 38.19123852234599070, 72.05501292736988717 ) ) ;
#9810=VERTEX_POINT ( 'NONE', #14653 ) ;
#9811=CARTESIAN_POINT ( 'NONE',  ( 37.31606138205700063, 43.19123852234599070, 73.55501292736987295 ) ) ;
#9813=EDGE_CURVE ( 'NONE', #3466, #17958, #16715, .T. ) ;
#9815=ORIENTED_EDGE ( 'NONE', *, *, #10975, .T. ) ;
#9822=DIRECTION ( 'NONE',  ( 1.000000000000000000, 0.000000000000000000, 0.000000000000000000 ) ) ;
#9825=LINE ( 'NONE', #13808, #13479 ) ;
#9826=EDGE_CURVE ( 'NONE', #21184, #3194, #15323, .T. ) ;
#9829=STYLED_ITEM ( 'NONE', ( #15447 ), #8398 ) ;
#9838=FACE_OUTER_BOUND ( 'NONE', #1434, .T. ) ;
#9843=ORIENTED_EDGE ( 'NONE', *, *, #245, .T. ) ;
#9849=DIRECTION ( 'NONE',  ( 0.000000000000000000, 1.000000000000000000, -2.999999999999999839E-15 ) ) ;
#9862=CARTESIAN_POINT ( 'NONE',  ( 44.81606138205700063, -36.55876147765400930, 73.30501292737011454 ) ) ;
#9870=VERTEX_POINT ( 'NONE', #6670 ) ;
#9873=EDGE_CURVE ( 'NONE', #10709, #6775, #18623, .T. ) ;
#9876=ORIENTED_EDGE ( 'NONE', *, *, #16568, .T. ) ;
#9879=CARTESIAN_POINT ( 'NONE',  ( 40.31606138205700773, 37.94123852234599070, 73.55501292736988717 ) ) ;
#9885=AXIS2_PLACEMENT_3D ( 'NONE', #5524, #25067, #3572 ) ;
#9891=ORIENTED_EDGE ( 'NONE', *, *, #16247, .T. ) ;
#9895=EDGE_CURVE ( 'NONE', #10392, #22023, #24433, .T. ) ;
#9903=CARTESIAN_POINT ( 'NONE',  ( 40.81606138205700773, 37.44123852234599781, 75.30501292736990138 ) ) ;
#9904=EDGE_LOOP ( 'NONE', ( #1511, #15818, #24424, #18178 ) ) ;
#9905=VERTEX_POINT ( 'NONE', #6932 ) ;
#9919=PLANE ( 'NONE',  #17391 ) ;
#9921=CARTESIAN_POINT ( 'NONE',  ( 36.31606138205700063, -31.05876147765399864, 74.30501292737010033 ) ) ;
#9924=DIRECTION ( 'NONE',  ( 0.000000000000000000, -1.000000000000000000, 2.999999999999999839E-15 ) ) ;
#9937=ORIENTED_EDGE ( 'NONE', *, *, #10147, .T. ) ;
#9943=DIRECTION ( 'NONE',  ( -1.000000000000000000, 0.000000000000000000, 0.000000000000000000 ) ) ;
#9958=DIRECTION ( 'NONE',  ( 0.000000000000000000, -1.000000000000000000, 3.325260651745651169E-15 ) ) ;
#9967=VERTEX_POINT ( 'NONE', #25186 ) ;
#9979=DIRECTION ( 'NONE',  ( 3.373073425510455500E-16, 2.999999999999999839E-15, 1.000000000000000000 ) ) ;
#9980=AXIS2_PLACEMENT_3D ( 'NONE', #11577, #11833, #1623 ) ;
#9984=DIRECTION ( 'NONE',  ( 0.000000000000000000, 1.000000000000000000, -2.913263826201159484E-15 ) ) ;
#9991=CARTESIAN_POINT ( 'NONE',  ( 40.81606138205700773, -24.05876147765399864, 75.30501292737008612 ) ) ;
#10008=ORIENTED_EDGE ( 'NONE', *, *, #22773, .F. ) ;
#10017=DIRECTION ( 'NONE',  ( -1.000000000000000000, 0.000000000000000000, 0.000000000000000000 ) ) ;
#10019=AXIS2_PLACEMENT_3D ( 'NONE', #944, #18992, #9220 ) ;
#10023=DIRECTION ( 'NONE',  ( -1.000000000000000000, 1.301042606982604506E-30, 4.336808689942015271E-16 ) ) ;
#10027=DIRECTION ( 'NONE',  ( -1.000000000000000000, 5.204170427930415223E-30, 1.734723475976805122E-15 ) ) ;
#10034=ORIENTED_EDGE ( 'NONE', *, *, #16044, .F. ) ;
#10035=PLANE ( 'NONE',  #22283 ) ;
#10038=ORIENTED_EDGE ( 'NONE', *, *, #13879, .T. ) ;
#10042=CARTESIAN_POINT ( 'NONE',  ( 40.81606138205700773, -24.05876147765399864, 75.30501292737008612 ) ) ;
#10050=AXIS2_PLACEMENT_3D ( 'NONE', #9720, #2093, #25276 ) ;
#10064=EDGE_CURVE ( 'NONE', #8849, #6796, #12899, .T. ) ;
#10071=ORIENTED_EDGE ( 'NONE', *, *, #4374, .F. ) ;
#10088=DIRECTION ( 'NONE',  ( 1.000000000000000000, -1.301042606982604506E-30, -4.336808689942015271E-16 ) ) ;
#10089=VECTOR ( 'NONE', #22693, 1000.000000000000000 ) ;
#10105=FACE_OUTER_BOUND ( 'NONE', #9757, .T. ) ;
#10115=ORIENTED_EDGE ( 'NONE', *, *, #9895, .F. ) ;
#10116=LINE ( 'NONE', #12307, #8184 ) ;
#10128=ORIENTED_EDGE ( 'NONE', *, *, #21241, .T. ) ;
#10135=EDGE_CURVE ( 'NONE', #8061, #10587, #18130, .T. ) ;
#10147=EDGE_CURVE ( 'NONE', #2806, #18113, #12082, .T. ) ;
#10153=ORIENTED_EDGE ( 'NONE', *, *, #7051, .F. ) ;
#10170=FACE_OUTER_BOUND ( 'NONE', #14492, .T. ) ;
#10171=LINE ( 'NONE', #18163, #5725 ) ;
#10173=ORIENTED_EDGE ( 'NONE', *, *, #16919, .T. ) ;
#10175=CARTESIAN_POINT ( 'NONE',  ( 38.31606138205700063, 38.69123852234597649, 69.30501292736988717 ) ) ;
#10182=EDGE_CURVE ( 'NONE', #25304, #19848, #10428, .T. ) ;
#10187=ORIENTED_EDGE ( 'NONE', *, *, #15205, .F. ) ;
#10188=DIRECTION ( 'NONE',  ( 1.734723475976804876E-16, 2.999999999999999839E-15, 1.000000000000000000 ) ) ;
#10189=DIRECTION ( 'NONE',  ( 0.000000000000000000, 1.000000000000000000, 0.000000000000000000 ) ) ;
#10193=EDGE_CURVE ( 'NONE', #3194, #14256, #8780, .T. ) ;
#10199=FACE_OUTER_BOUND ( 'NONE', #13504, .T. ) ;
#10200=EDGE_CURVE ( 'NONE', #10286, #20311, #24031, .T. ) ;
#10204=CARTESIAN_POINT ( 'NONE',  ( 32.81606138205700773, -34.55876147765401640, 70.30501292737011454 ) ) ;
#10215=ORIENTED_EDGE ( 'NONE', *, *, #21070, .T. ) ;
#10216=PLANE ( 'NONE',  #11119 ) ;
#10227=PLANE ( 'NONE',  #19817 ) ;
#10230=ORIENTED_EDGE ( 'NONE', *, *, #4462, .F. ) ;
#10257=CARTESIAN_POINT ( 'NONE',  ( 35.81606138205700063, -24.05876147765399864, 75.30501292737008612 ) ) ;
#10264=ORIENTED_EDGE ( 'NONE', *, *, #2727, .F. ) ;
#10265=AXIS2_PLACEMENT_3D ( 'NONE', #1155, #9047, #22812 ) ;
#10278=ADVANCED_FACE ( 'NONE', ( #78, #4089 ), #11961, .T. ) ;
#10279=CIRCLE ( 'NONE', #13564, 1.000000000000000888 ) ;
#10286=VERTEX_POINT ( 'NONE', #22485 ) ;
#10290=LINE ( 'NONE', #23925, #4237 ) ;
#10294=LINE ( 'NONE', #6547, #20145 ) ;
#10305=DIRECTION ( 'NONE',  ( 1.000000000000000000, -9.027796614315171564E-31, -4.436993566807132493E-46 ) ) ;
#10308=UNCERTAINTY_MEASURE_WITH_UNIT (LENGTH_MEASURE( 1.000000000000000082E-05 ), #13225, 'distance_accuracy_value', 'NONE');
#10309=CIRCLE ( 'NONE', #4151, 1.750000000000001554 ) ;
#10322=DIRECTION ( 'NONE',  ( -1.000000000000000000, 1.115179377413661005E-30, 3.717264591378870232E-16 ) ) ;
#10323=AXIS2_PLACEMENT_3D ( 'NONE', #21779, #20094, #2560 ) ;
#10335=CARTESIAN_POINT ( 'NONE',  ( 32.81606138205700773, -33.00876147765401925, 70.30501292737011454 ) ) ;
#10345=ORIENTED_EDGE ( 'NONE', *, *, #10359, .F. ) ;
#10346=PLANE ( 'NONE',  #22822 ) ;
#10358=EDGE_CURVE ( 'NONE', #6560, #15661, #12712, .T. ) ;
#10359=EDGE_CURVE ( 'NONE', #21318, #9870, #8370, .T. ) ;
#10392=VERTEX_POINT ( 'NONE', #14505 ) ;
#10397=CARTESIAN_POINT ( 'NONE',  ( 32.81606138205700773, 32.99511671078946762, 63.14259751872857152 ) ) ;
#10408=CARTESIAN_POINT ( 'NONE',  ( 31.81606138205700418, -33.00876147765401925, 70.30501292737011454 ) ) ;
#10420=VECTOR ( 'NONE', #4973, 1000.000000000000000 ) ;
#10423=EDGE_CURVE ( 'NONE', #19848, #6622, #2888, .T. ) ;
#10428=CIRCLE ( 'NONE', #24801, 1.000000000000000888 ) ;
#10444=CARTESIAN_POINT ( 'NONE',  ( 32.81606138205700773, 28.12806996228107437, 66.30501292736992980 ) ) ;
#10458=DIRECTION ( 'NONE',  ( -6.938893903907229955E-15, -1.000000000000000000, 3.000000000000000628E-15 ) ) ;
#10459=VECTOR ( 'NONE', #20481, 1000.000000000000000 ) ;
#10464=VERTEX_POINT ( 'NONE', #22988 ) ;
#10485=CARTESIAN_POINT ( 'NONE',  ( 43.81606138205700063, -34.55876147765400930, 73.30501292737011454 ) ) ;
#10498=CARTESIAN_POINT ( 'NONE',  ( 35.81606138205700063, -31.05876147765399864, 75.30501292737010033 ) ) ;
#10505=DIRECTION ( 'NONE',  ( 0.000000000000000000, 3.469446951953611033E-15, 1.000000000000000000 ) ) ;
#10506=DIRECTION ( 'NONE',  ( -1.000000000000000000, 3.083952846180990083E-15, -9.251858538542970050E-30 ) ) ;
#10510=ORIENTED_EDGE ( 'NONE', *, *, #7509, .T. ) ;
#10512=LINE ( 'NONE', #22353, #23132 ) ;
#10517=DIRECTION ( 'NONE',  ( 1.000000000000000000, 0.000000000000000000, 0.000000000000000000 ) ) ;
#10520=EDGE_CURVE ( 'NONE', #1727, #15791, #24902, .T. ) ;
#10533=EDGE_CURVE ( 'NONE', #1877, #13391, #17012, .T. ) ;
#10537=ORIENTED_EDGE ( 'NONE', *, *, #12413, .T. ) ;
#10542=ORIENTED_EDGE ( 'NONE', *, *, #6590, .F. ) ;
#10551=VECTOR ( 'NONE', #9297, 1000.000000000000114 ) ;
#10557=DIRECTION ( 'NONE',  ( 0.000000000000000000, 2.999999999999999839E-15, 1.000000000000000000 ) ) ;
#10569=ORIENTED_EDGE ( 'NONE', *, *, #4361, .F. ) ;
#10575=FACE_OUTER_BOUND ( 'NONE', #3636, .T. ) ;
#10587=VERTEX_POINT ( 'NONE', #15262 ) ;
#10591=CARTESIAN_POINT ( 'NONE',  ( 44.81606138205700063, -36.55876147765401640, 71.30501292737011454 ) ) ;
#10597=VERTEX_POINT ( 'NONE', #21696 ) ;
#10605=CARTESIAN_POINT ( 'NONE',  ( 44.81606138205700063, 41.44123852234599781, 75.30501292736987295 ) ) ;
#10608=DIRECTION ( 'NONE',  ( 0.000000000000000000, -1.000000000000000000, 2.999999999999999839E-15 ) ) ;
#10612=CARTESIAN_POINT ( 'NONE',  ( 44.81606138205700063, -34.55876147765400930, 73.30501292737011454 ) ) ;
#10613=VECTOR ( 'NONE', #22824, 1000.000000000000000 ) ;
#10616=VECTOR ( 'NONE', #23906, 1000.000000000000000 ) ;
#10621=CARTESIAN_POINT ( 'NONE',  ( 40.81606138205700773, -31.05876147765399864, 74.30501292737010033 ) ) ;
#10626=ORIENTED_EDGE ( 'NONE', *, *, #10533, .F. ) ;
#10630=CIRCLE ( 'NONE', #22531, 1.750000000000001554 ) ;
#10634=AXIS2_PLACEMENT_3D ( 'NONE', #6857, #5061, #13052 ) ;
#10637=ORIENTED_EDGE ( 'NONE', *, *, #6581, .T. ) ;
#10639=CARTESIAN_POINT ( 'NONE',  ( 31.81606138205700418, -38.55876147765401640, 71.30501292737012875 ) ) ;
#10647=VERTEX_POINT ( 'NONE', #8050 ) ;
#10648=ORIENTED_EDGE ( 'NONE', *, *, #4712, .F. ) ;
#10659=CARTESIAN_POINT ( 'NONE',  ( 31.81606138205700418, 1.441238522345976714, 67.80501292737001506 ) ) ;
#10661=EDGE_CURVE ( 'NONE', #23038, #21084, #4435, .T. ) ;
#10663=EDGE_LOOP ( 'NONE', ( #8987, #9684, #22145, #2895 ) ) ;
#10671=ORIENTED_EDGE ( 'NONE', *, *, #13965, .F. ) ;
#10675=VECTOR ( 'NONE', #20152, 1000.000000000000000 ) ;
#10683=DIRECTION ( 'NONE',  ( -0.000000000000000000, -1.000000000000000000, 2.848211695852029218E-15 ) ) ;
#10687=DIRECTION ( 'NONE',  ( 0.000000000000000000, 1.000000000000000000, -2.999999999999999839E-15 ) ) ;
#10692=LINE ( 'NONE', #5008, #15246 ) ;
#10693=ORIENTED_EDGE ( 'NONE', *, *, #15972, .F. ) ;
#10705=LINE ( 'NONE', #14806, #20375 ) ;
#10709=VERTEX_POINT ( 'NONE', #18217 ) ;
#10714=AXIS2_PLACEMENT_3D ( 'NONE', #9434, #17667, #21397 ) ;
#10731=VECTOR ( 'NONE', #23511, 1000.000000000000000 ) ;
#10741=CYLINDRICAL_SURFACE ( 'NONE', #20445, 1.750000000000001554 ) ;
#10745=LINE ( 'NONE', #9921, #19479 ) ;
#10771=DIRECTION ( 'NONE',  ( -8.673617379884039170E-17, 1.163336342344340343E-15, -1.000000000000000000 ) ) ;
#10780=LINE ( 'NONE', #24664, #2037 ) ;
#10802=CARTESIAN_POINT ( 'NONE',  ( 31.81606138205700418, 38.19123852234599070, 73.05501292736988717 ) ) ;
#10805=CIRCLE ( 'NONE', #19851, 2.500000000000002220 ) ;
#10807=ORIENTED_EDGE ( 'NONE', *, *, #16571, .T. ) ;
#10808=CARTESIAN_POINT ( 'NONE',  ( 43.81606138205700063, 41.44123852234599070, 73.55501292736987295 ) ) ;
#10810=EDGE_CURVE ( 'NONE', #17954, #1877, #8933, .T. ) ;
#10812=ORIENTED_EDGE ( 'NONE', *, *, #5948, .T. ) ;
#10816=AXIS2_PLACEMENT_3D ( 'NONE', #24257, #6128, #22215 ) ;
#10818=CARTESIAN_POINT ( 'NONE',  ( 40.81606138205700773, -24.05876147765400219, 74.30501292737008612 ) ) ;
#10821=ORIENTED_EDGE ( 'NONE', *, *, #6900, .T. ) ;
#10827=EDGE_CURVE ( 'NONE', #23038, #25254, #16269, .T. ) ;
#10828=LINE ( 'NONE', #17008, #1173 ) ;
#10833=VECTOR ( 'NONE', #12995, 1000.000000000000114 ) ;
#10837=EDGE_CURVE ( 'NONE', #11585, #22327, #9210, .T. ) ;
#10847=ADVANCED_FACE ( 'NONE', ( #14845 ), #22703, .T. ) ;
#10849=DIRECTION ( 'NONE',  ( -1.000000000000000000, 0.000000000000000000, 0.000000000000000000 ) ) ;
#10857=CARTESIAN_POINT ( 'NONE',  ( 31.81606138205700418, 41.44123852234599781, 75.30501292736988717 ) ) ;
#10858=EDGE_CURVE ( 'NONE', #1424, #13483, #14346, .T. ) ;
#10860=CYLINDRICAL_SURFACE ( 'NONE', #13781, 0.7500000000000006661 ) ;
#10864=DIRECTION ( 'NONE',  ( 1.734723475976804876E-16, -1.163336342344340343E-15, 1.000000000000000000 ) ) ;
#10869=LINE ( 'NONE', #10612, #14320 ) ;
#10876=CARTESIAN_POINT ( 'NONE',  ( 32.81606138205700773, 28.12806996228107081, 65.30501292736992980 ) ) ;
#10877=VECTOR ( 'NONE', #16932, 1000.000000000000000 ) ;
#10882=ORIENTED_EDGE ( 'NONE', *, *, #3161, .F. ) ;
#10903=ORIENTED_EDGE ( 'NONE', *, *, #9895, .T. ) ;
#10906=FACE_OUTER_BOUND ( 'NONE', #23813, .T. ) ;
#10913=ORIENTED_EDGE ( 'NONE', *, *, #4063, .T. ) ;
#10919=EDGE_CURVE ( 'NONE', #16707, #10709, #10745, .T. ) ;
#10929=CYLINDRICAL_SURFACE ( 'NONE', #1006, 1.000000000000000888 ) ;
#10930=CARTESIAN_POINT ( 'NONE',  ( 43.81606138205700063, 39.55420052130484265, 58.58767820587064534 ) ) ;
#10936=CARTESIAN_POINT ( 'NONE',  ( 31.81606138205700418, 38.19123852234598360, 71.05501292736988717 ) ) ;
#10945=PLANE ( 'NONE',  #4149 ) ;
#10954=DIRECTION ( 'NONE',  ( 1.000000000000000000, -1.301042606982604506E-30, -4.336808689942015271E-16 ) ) ;
#10957=EDGE_CURVE ( 'NONE', #5909, #23734, #17048, .T. ) ;
#10967=EDGE_CURVE ( 'NONE', #13165, #14979, #21633, .T. ) ;
#10975=EDGE_CURVE ( 'NONE', #10597, #17161, #19436, .T. ) ;
#10988=ADVANCED_FACE ( 'NONE', ( #5922 ), #7862, .T. ) ;
#10989=DIRECTION ( 'NONE',  ( 3.717264591378870232E-16, 3.129456975819164530E-15, 1.000000000000000000 ) ) ;
#10990=VERTEX_POINT ( 'NONE', #3244 ) ;
#10999=DIRECTION ( 'NONE',  ( 0.000000000000000000, 1.000000000000000000, -1.387778780781444413E-14 ) ) ;
#11004=ORIENTED_EDGE ( 'NONE', *, *, #24176, .F. ) ;
#11008=EDGE_CURVE ( 'NONE', #1424, #1244, #1390, .T. ) ;
#11012=LINE ( 'NONE', #24891, #986 ) ;
#11027=LINE ( 'NONE', #3028, #10420 ) ;
#11040=CARTESIAN_POINT ( 'NONE',  ( 35.31606138205687273, 43.19123852234596939, 65.30501292736988717 ) ) ;
#11041=CARTESIAN_POINT ( 'NONE',  ( 43.06606138205700063, -34.55876147765400930, 73.55501292737011454 ) ) ;
#11056=AXIS2_PLACEMENT_3D ( 'NONE', #6428, #8365, #8104 ) ;
#11058=ADVANCED_FACE ( 'NONE', ( #3378 ), #15100, .F. ) ;
#11059=CARTESIAN_POINT ( 'NONE',  ( 33.56606138205700773, -38.55876147765400930, 73.55501292737012875 ) ) ;
#11061=ADVANCED_FACE ( 'NONE', ( #9202 ), #21037, .F. ) ;
#11065=CYLINDRICAL_SURFACE ( 'NONE', #9885, 0.7500000000000006661 ) ;
#11074=DIRECTION ( 'NONE',  ( -1.000000000000000000, 6.195440985631514482E-17, 1.836970198721027715E-16 ) ) ;
#11080=LINE ( 'NONE', #12638, #16660 ) ;
#11083=EDGE_LOOP ( 'NONE', ( #4764, #21183, #14960, #24914, #23262, #8583, #7480, #24883, #24835, #23101, #16129 ) ) ;
#11106=VERTEX_POINT ( 'NONE', #738 ) ;
#11109=CIRCLE ( 'NONE', #14395, 0.5000000000000004441 ) ;
#11110=DIRECTION ( 'NONE',  ( 1.000000000000000000, 0.000000000000000000, 0.000000000000000000 ) ) ;
#11119=AXIS2_PLACEMENT_3D ( 'NONE', #8415, #16126, #24221 ) ;
#11124=DIRECTION ( 'NONE',  ( 0.000000000000000000, -1.000000000000000000, 2.999999999999999839E-15 ) ) ;
#11139=DIRECTION ( 'NONE',  ( 0.000000000000000000, -2.999999999999999839E-15, -1.000000000000000000 ) ) ;
#11144=ORIENTED_EDGE ( 'NONE', *, *, #20763, .T. ) ;
#11145=DIRECTION ( 'NONE',  ( -1.000000000000000000, 1.115179377413661005E-30, 3.717264591378870232E-16 ) ) ;
#11158=DIRECTION ( 'NONE',  ( 0.000000000000000000, -1.000000000000000000, 2.999999999999999839E-15 ) ) ;
#11160=CARTESIAN_POINT ( 'NONE',  ( 40.31606138205700773, 37.94123852234599781, 74.30501292736988717 ) ) ;
#11161=VECTOR ( 'NONE', #22243, 1000.000000000000000 ) ;
#11171=EDGE_CURVE ( 'NONE', #22563, #24485, #24175, .T. ) ;
#11189=ORIENTED_EDGE ( 'NONE', *, *, #5389, .F. ) ;
#11190=ORIENTED_EDGE ( 'NONE', *, *, #19159, .T. ) ;
#11191=DIRECTION ( 'NONE',  ( 0.000000000000000000, 1.000000000000000000, 0.000000000000000000 ) ) ;
#11199=VERTEX_POINT ( 'NONE', #20208 ) ;
#11216=AXIS2_PLACEMENT_3D ( 'NONE', #5634, #13383, #19286 ) ;
#11239=EDGE_LOOP ( 'NONE', ( #19146, #8792, #19461, #19501 ) ) ;
#11245=ORIENTED_EDGE ( 'NONE', *, *, #5363, .T. ) ;
#11246=AXIS2_PLACEMENT_3D ( 'NONE', #16816, #20687, #24402 ) ;
#11257=CARTESIAN_POINT ( 'NONE',  ( 33.56606138205700773, 41.44123852234595518, 61.30501292736988006 ) ) ;
#11264=CARTESIAN_POINT ( 'NONE',  ( 40.31606138205700773, 37.94123852234599070, 73.55501292736988717 ) ) ;
#11289=CARTESIAN_POINT ( 'NONE',  ( 43.06606138205700063, 43.19123852234601202, 79.18605660143489899 ) ) ;
#11297=AXIS2_PLACEMENT_3D ( 'NONE', #18239, #24128, #12066 ) ;
#11307=EDGE_LOOP ( 'NONE', ( #14805, #3905, #13914, #948, #4916, #23568, #24044, #6519, #4586, #8298, #3207, #4983 ) ) ;
#11311=EDGE_CURVE ( 'NONE', #23735, #1877, #20977, .T. ) ;
#11315=CARTESIAN_POINT ( 'NONE',  ( 43.06606138205700063, -38.55876147765400219, 74.30501292737012875 ) ) ;
#11320=ADVANCED_FACE ( 'NONE', ( #12621 ), #9269, .F. ) ;
#11332=EDGE_LOOP ( 'NONE', ( #16466, #16033, #22361, #325 ) ) ;
#11333=CARTESIAN_POINT ( 'NONE',  ( 31.81606138205700418, 18.19123852234599070, 72.05501292736995822 ) ) ;
#11335=ORIENTED_EDGE ( 'NONE', *, *, #3112, .T. ) ;
#11336=ORIENTED_EDGE ( 'NONE', *, *, #10193, .F. ) ;
#11343=CARTESIAN_POINT ( 'NONE',  ( 43.06606138205700063, 41.44123852234599070, 73.55501292736987295 ) ) ;
#11345=AXIS2_PLACEMENT_3D ( 'NONE', #1405, #22794, #20611 ) ;
#11349=FACE_OUTER_BOUND ( 'NONE', #15379, .T. ) ;
#11354=ORIENTED_EDGE ( 'NONE', *, *, #24838, .F. ) ;
#11365=FACE_BOUND ( 'NONE', #8718, .T. ) ;
#11368=VERTEX_POINT ( 'NONE', #16718 ) ;
#11369=DIRECTION ( 'NONE',  ( -1.000000000000000000, 1.115179377413661005E-30, 3.717264591378870232E-16 ) ) ;
#11377=ORIENTED_EDGE ( 'NONE', *, *, #20927, .T. ) ;
#11408=AXIS2_PLACEMENT_3D ( 'NONE', #3787, #11671, #19512 ) ;
#11423=ORIENTED_EDGE ( 'NONE', *, *, #10919, .T. ) ;
#11428=VECTOR ( 'NONE', #737, 1000.000000000000000 ) ;
#11431=ORIENTED_EDGE ( 'NONE', *, *, #22943, .T. ) ;
#11432=ADVANCED_FACE ( 'NONE', ( #24688 ), #7062, .F. ) ;
#11440=EDGE_LOOP ( 'NONE', ( #12790, #8482, #17514, #22656 ) ) ;
#11446=EDGE_CURVE ( 'NONE', #24313, #14570, #17797, .T. ) ;
#11452=DIRECTION ( 'NONE',  ( 1.000000000000000000, 0.000000000000000000, 0.000000000000000000 ) ) ;
#11455=CARTESIAN_POINT ( 'NONE',  ( 38.31606138205687984, 43.19123852234599781, 75.30501292736987295 ) ) ;
#11461=DIRECTION ( 'NONE',  ( 1.000000000000000000, 3.083952846180990083E-15, -9.251858538542970050E-30 ) ) ;
#11463=CIRCLE ( 'NONE', #4062, 0.5000000000000004441 ) ;
#11467=CARTESIAN_POINT ( 'NONE',  ( 31.81606138205700418, 38.19123852234599070, 73.05501292736988717 ) ) ;
#11476=ADVANCED_FACE ( 'NONE', ( #3694 ), #17361, .F. ) ;
#11477=CARTESIAN_POINT ( 'NONE',  ( 43.81606138205700063, -38.55876147765401640, 71.30501292737012875 ) ) ;
#11497=ORIENTED_EDGE ( 'NONE', *, *, #7716, .F. ) ;
#11498=LINE ( 'NONE', #17545, #12982 ) ;
#11499=DIRECTION ( 'NONE',  ( -3.854941057726235139E-16, -2.999999999999999839E-15, -1.000000000000000000 ) ) ;
#11509=LINE ( 'NONE', #17553, #3590 ) ;
#11525=DIRECTION ( 'NONE',  ( 0.000000000000000000, -3.469446951953611033E-15, 1.000000000000000000 ) ) ;
#11536=EDGE_CURVE ( 'NONE', #22091, #21703, #21501, .T. ) ;
#11558=DIRECTION ( 'NONE',  ( -1.000000000000000000, 1.115179377413661005E-30, 3.717264591378870232E-16 ) ) ;
#11566=LINE ( 'NONE', #19404, #12813 ) ;
#11569=EDGE_CURVE ( 'NONE', #17699, #17085, #19671, .T. ) ;
#11577=CARTESIAN_POINT ( 'NONE',  ( 43.81606138205700063, 28.12806996228107081, 65.30501292736992980 ) ) ;
#11585=VERTEX_POINT ( 'NONE', #25324 ) ;
#11596=DIRECTION ( 'NONE',  ( 0.000000000000000000, 1.000000000000000000, -2.999999999999999839E-15 ) ) ;
#11598=LINE ( 'NONE', #21249, #7933 ) ;
#11609=ORIENTED_EDGE ( 'NONE', *, *, #6906, .T. ) ;
#11614=ORIENTED_EDGE ( 'NONE', *, *, #5799, .F. ) ;
#11626=ADVANCED_FACE ( 'NONE', ( #6022 ), #22109, .T. ) ;
#11628=ADVANCED_FACE ( 'NONE', ( #21990, #20055, #23784, #24036 ), #4599, .T. ) ;
#11635=EDGE_CURVE ( 'NONE', #13053, #10990, #14138, .T. ) ;
#11654=DIRECTION ( 'NONE',  ( 0.000000000000000000, -1.000000000000000000, 0.000000000000000000 ) ) ;
#11658=LINE ( 'NONE', #17832, #6356 ) ;
#11671=DIRECTION ( 'NONE',  ( 0.000000000000000000, -2.999999999999999839E-15, -1.000000000000000000 ) ) ;
#11678=VECTOR ( 'NONE', #14722, 1000.000000000000000 ) ;
#11685=CARTESIAN_POINT ( 'NONE',  ( 34.81606138205687273, 33.19123852234595518, 61.80501292736990848 ) ) ;
#11689=FACE_OUTER_BOUND ( 'NONE', #1074, .T. ) ;
#11703=CIRCLE ( 'NONE', #555, 1.000000000000000888 ) ;
#11709=DIRECTION ( 'NONE',  ( 1.000000000000000000, 0.000000000000000000, 0.000000000000000000 ) ) ;
#11723=CYLINDRICAL_SURFACE ( 'NONE', #7487, 2.500000000000002220 ) ;
#11727=CARTESIAN_POINT ( 'NONE',  ( 40.81606138205700773, 37.44123852234599781, 75.30501292736990138 ) ) ;
#11728=LINE ( 'NONE', #9535, #23182 ) ;
#11729=EDGE_CURVE ( 'NONE', #2388, #3119, #1751, .T. ) ;
#11745=VERTEX_POINT ( 'NONE', #19933 ) ;
#11756=DIRECTION ( 'NONE',  ( 0.000000000000000000, 1.000000000000000000, -2.999999999999999839E-15 ) ) ;
#11757=CARTESIAN_POINT ( 'NONE',  ( 40.81606138205700773, 37.44123852234599781, 74.30501292736988717 ) ) ;
#11777=ORIENTED_EDGE ( 'NONE', *, *, #23995, .F. ) ;
#11788=LINE ( 'NONE', #10444, #9009 ) ;
#11795=APPLICATION_CONTEXT ( 'automotive_design' ) ;
#11797=LINE ( 'NONE', #7544, #21673 ) ;
#11800=VERTEX_POINT ( 'NONE', #5110 ) ;
#11808=DIRECTION ( 'NONE',  ( 0.000000000000000000, -1.000000000000000000, 2.999999999999999839E-15 ) ) ;
#11819=EDGE_CURVE ( 'NONE', #8848, #9377, #11027, .T. ) ;
#11820=LINE ( 'NONE', #5883, #3746 ) ;
#11823=VECTOR ( 'NONE', #268, 1000.000000000000000 ) ;
#11831=EDGE_CURVE ( 'NONE', #16347, #22563, #20559, .T. ) ;
#11833=DIRECTION ( 'NONE',  ( -1.000000000000000000, 0.000000000000000000, 0.000000000000000000 ) ) ;
#11848=VERTEX_POINT ( 'NONE', #16558 ) ;
#11854=ADVANCED_FACE ( 'NONE', ( #10906 ), #3286, .T. ) ;
#11869=DIRECTION ( 'NONE',  ( 0.000000000000000000, 0.000000000000000000, 1.000000000000000000 ) ) ;
#11871=AXIS2_PLACEMENT_3D ( 'NONE', #4514, #14185, #8256 ) ;
#11877=ORIENTED_EDGE ( 'NONE', *, *, #1826, .T. ) ;
#11895=ADVANCED_FACE ( 'NONE', ( #6783 ), #2893, .T. ) ;
#11908=ORIENTED_EDGE ( 'NONE', *, *, #22789, .F. ) ;
#11918=ORIENTED_EDGE ( 'NONE', *, *, #14980, .T. ) ;
#11919=VECTOR ( 'NONE', #12123, 1000.000000000000000 ) ;
#11924=( LENGTH_UNIT ( ) NAMED_UNIT ( * ) SI_UNIT ( .MILLI., .METRE. ) );
#11925=CARTESIAN_POINT ( 'NONE',  ( 32.81606138205700773, -24.55876147765400574, 72.80501292737008612 ) ) ;
#11929=EDGE_CURVE ( 'NONE', #15369, #22901, #6904, .T. ) ;
#11937=LINE ( 'NONE', #18111, #18969 ) ;
#11938=ORIENTED_EDGE ( 'NONE', *, *, #11008, .F. ) ;
#11941=CIRCLE ( 'NONE', #2832, 1.550000000000002709 ) ;
#11961=PLANE ( 'NONE',  #14128 ) ;
#11964=PLANE ( 'NONE',  #1966 ) ;
#11970=ADVANCED_FACE ( 'NONE', ( #19382 ), #5863, .T. ) ;
#11973=EDGE_LOOP ( 'NONE', ( #2161, #4579, #13763, #8789 ) ) ;
#11978=CIRCLE ( 'NONE', #21003, 2.500000000000002220 ) ;
#11980=EDGE_CURVE ( 'NONE', #19667, #4130, #13722, .T. ) ;
#11983=VECTOR ( 'NONE', #24311, 1000.000000000000000 ) ;
#11990=EDGE_LOOP ( 'NONE', ( #16860, #13892, #24196, #11377 ) ) ;
#11991=CARTESIAN_POINT ( 'NONE',  ( 43.81606138205700063, 41.44123852234595518, 61.30501292736988006 ) ) ;
#12006=CARTESIAN_POINT ( 'NONE',  ( 31.81606138205700418, -34.55876147765401640, 70.30501292737011454 ) ) ;
#12013=VECTOR ( 'NONE', #15535, 1000.000000000000000 ) ;
#12029=CARTESIAN_POINT ( 'NONE',  ( 40.31606138205700773, 37.94123852234599781, 75.30501292736988717 ) ) ;
#12037=VERTEX_POINT ( 'NONE', #25415 ) ;
#12046=AXIS2_PLACEMENT_3D ( 'NONE', #12341, #8592, #20317 ) ;
#12048=ORIENTED_EDGE ( 'NONE', *, *, #5750, .F. ) ;
#12051=VECTOR ( 'NONE', #824, 1000.000000000000000 ) ;
#12053=PLANE ( 'NONE',  #14137 ) ;
#12057=VECTOR ( 'NONE', #3050, 1000.000000000000000 ) ;
#12058=CARTESIAN_POINT ( 'NONE',  ( 43.81606138205700063, -34.55876147765401640, 70.30501292737011454 ) ) ;
#12060=DIRECTION ( 'NONE',  ( 1.000000000000000000, 1.115287202090205222E-30, -1.734723475976805122E-15 ) ) ;
#12065=VECTOR ( 'NONE', #3660, 1000.000000000000000 ) ;
#12066=DIRECTION ( 'NONE',  ( 1.000000000000000000, 0.000000000000000000, 0.000000000000000000 ) ) ;
#12071=LINE ( 'NONE', #23770, #10731 ) ;
#12073=FACE_OUTER_BOUND ( 'NONE', #3774, .T. ) ;
#12078=EDGE_CURVE ( 'NONE', #20194, #4468, #6301, .T. ) ;
#12082=LINE ( 'NONE', #4471, #7956 ) ;
#12086=CIRCLE ( 'NONE', #12512, 4.000000000000003553 ) ;
#12094=ORIENTED_EDGE ( 'NONE', *, *, #24060, .F. ) ;
#12097=DIRECTION ( 'NONE',  ( 5.664403186863039509E-16, 3.000000000000000628E-15, 1.000000000000000000 ) ) ;
#12103=EDGE_CURVE ( 'NONE', #7176, #1142, #7671, .T. ) ;
#12123=DIRECTION ( 'NONE',  ( 1.000000000000000000, 0.000000000000000000, 0.000000000000000000 ) ) ;
#12137=DIRECTION ( 'NONE',  ( -1.000000000000000000, 6.938893903907231533E-15, 6.505213034912821500E-16 ) ) ;
#12138=VERTEX_POINT ( 'NONE', #11925 ) ;
#12140=DIRECTION ( 'NONE',  ( 1.000000000000000000, 0.000000000000000000, 0.000000000000000000 ) ) ;
#12141=ADVANCED_FACE ( 'NONE', ( #13845 ), #22203, .F. ) ;
#12143=AXIS2_PLACEMENT_3D ( 'NONE', #8924, #17162, #16768 ) ;
#12151=ADVANCED_FACE ( 'NONE', ( #16144 ), #2239, .F. ) ;
#12182=CARTESIAN_POINT ( 'NONE',  ( 31.81606138205700418, 38.19123852234598360, 71.05501292736988717 ) ) ;
#12188=VERTEX_POINT ( 'NONE', #21825 ) ;
#12194=CYLINDRICAL_SURFACE ( 'NONE', #16619, 1.000000000000000888 ) ;
#12199=LINE ( 'NONE', #12454, #9108 ) ;
#12201=DIRECTION ( 'NONE',  ( 0.000000000000000000, -2.999999999999999839E-15, -1.000000000000000000 ) ) ;
#12204=LINE ( 'NONE', #14129, #4002 ) ;
#12208=DIRECTION ( 'NONE',  ( 1.000000000000000000, 0.000000000000000000, 0.000000000000000000 ) ) ;
#12228=EDGE_CURVE ( 'NONE', #15455, #17954, #15895, .T. ) ;
#12237=VECTOR ( 'NONE', #17308, 1000.000000000000000 ) ;
#12257=CARTESIAN_POINT ( 'NONE',  ( 36.31606138205700063, 41.44123852234599781, 75.30501292736987295 ) ) ;
#12259=ADVANCED_FACE ( 'NONE', ( #17972 ), #12053, .F. ) ;
#12267=EDGE_CURVE ( 'NONE', #11848, #9810, #23633, .T. ) ;
#12276=DIRECTION ( 'NONE',  ( -1.000000000000000000, 0.000000000000000000, 0.000000000000000000 ) ) ;
#12277=ADVANCED_FACE ( 'NONE', ( #4805 ), #2992, .T. ) ;
#12289=EDGE_CURVE ( 'NONE', #4665, #2525, #540, .T. ) ;
#12304=SURFACE_STYLE_FILL_AREA ( #19899 ) ;
#12307=CARTESIAN_POINT ( 'NONE',  ( 40.31606138205700773, -31.05876147765399864, 74.30501292737010033 ) ) ;
#12320=VECTOR ( 'NONE', #20210, 1000.000000000000000 ) ;
#12327=LINE ( 'NONE', #18247, #20272 ) ;
#12331=VECTOR ( 'NONE', #20765, 1000.000000000000000 ) ;
#12332=CARTESIAN_POINT ( 'NONE',  ( 43.81606138205700063, 38.19123852234599070, 73.05501292736988717 ) ) ;
#12336=AXIS2_PLACEMENT_3D ( 'NONE', #19604, #10088, #14070 ) ;
#12340=CARTESIAN_POINT ( 'NONE',  ( 39.31606138205700063, 43.19123852234599070, 73.55501292736987295 ) ) ;
#12341=CARTESIAN_POINT ( 'NONE',  ( 38.31606138205712853, 42.19123852234599781, 75.30501292736987295 ) ) ;
#12349=CARTESIAN_POINT ( 'NONE',  ( 31.81606138205700418, -24.55876147765400574, 72.80501292737008612 ) ) ;
#12373=PLANE ( 'NONE',  #6139 ) ;
#12379=EDGE_LOOP ( 'NONE', ( #17093, #324, #19153, #364 ) ) ;
#12383=CARTESIAN_POINT ( 'NONE',  ( 32.81606138205700773, 39.19123852234599070, 72.05501292736988717 ) ) ;
#12388=CARTESIAN_POINT ( 'NONE',  ( 32.81606138205700773, 18.19123852234599070, 72.05501292736995822 ) ) ;
#12413=EDGE_CURVE ( 'NONE', #8243, #11199, #22709, .T. ) ;
#12414=DIRECTION ( 'NONE',  ( -1.000000000000000000, 0.000000000000000000, 0.000000000000000000 ) ) ;
#12417=EDGE_CURVE ( 'NONE', #25304, #3155, #22583, .T. ) ;
#12421=CARTESIAN_POINT ( 'NONE',  ( 43.06606138205700063, 42.19123852234601202, 79.18605660143489899 ) ) ;
#12422=CARTESIAN_POINT ( 'NONE',  ( 34.81606138205687273, 42.19123852234595518, 61.30501292736988006 ) ) ;
#12437=DIRECTION ( 'NONE',  ( -1.000000000000000000, 0.000000000000000000, 0.000000000000000000 ) ) ;
#12443=DIRECTION ( 'NONE',  ( 4.542565983319590233E-31, 1.000000000000000000, -2.999999999999999839E-15 ) ) ;
#12447=ORIENTED_EDGE ( 'NONE', *, *, #5771, .F. ) ;
#12454=CARTESIAN_POINT ( 'NONE',  ( 43.81606138205700063, 41.44123852234597649, 68.80501292736988717 ) ) ;
#12465=ORIENTED_EDGE ( 'NONE', *, *, #6948, .T. ) ;
#12469=AXIS2_PLACEMENT_3D ( 'NONE', #7606, #25085, #15449 ) ;
#12485=ORIENTED_EDGE ( 'NONE', *, *, #15855, .F. ) ;
#12487=ORIENTED_EDGE ( 'NONE', *, *, #13372, .T. ) ;
#12501=EDGE_CURVE ( 'NONE', #6757, #17565, #9219, .T. ) ;
#12512=AXIS2_PLACEMENT_3D ( 'NONE', #10204, #19990, #19864 ) ;
#12519=ORIENTED_EDGE ( 'NONE', *, *, #4909, .T. ) ;
#12525=PLANE ( 'NONE',  #4187 ) ;
#12546=CARTESIAN_POINT ( 'NONE',  ( 37.31606138205700063, 42.19123852234599781, 75.30501292736987295 ) ) ;
#12549=CARTESIAN_POINT ( 'NONE',  ( 44.81606138205700063, 35.38401127291550097, 61.48364296169660292 ) ) ;
#12551=CARTESIAN_POINT ( 'NONE',  ( 40.81606138205700773, 37.44123852234599781, 75.30501292736990138 ) ) ;
#12555=DIRECTION ( 'NONE',  ( 0.000000000000000000, 1.000000000000000000, -2.999999999999999839E-15 ) ) ;
#12573=ORIENTED_EDGE ( 'NONE', *, *, #17282, .F. ) ;
#12577=EDGE_LOOP ( 'NONE', ( #16668, #23627 ) ) ;
#12584=ORIENTED_EDGE ( 'NONE', *, *, #22873, .F. ) ;
#12589=DIRECTION ( 'NONE',  ( 0.000000000000000000, -1.000000000000000000, 2.999999999999999839E-15 ) ) ;
#12604=FACE_OUTER_BOUND ( 'NONE', #2831, .T. ) ;
#12621=FACE_OUTER_BOUND ( 'NONE', #10663, .T. ) ;
#12625=PLANE ( 'NONE',  #23830 ) ;
#12634=EDGE_CURVE ( 'NONE', #4199, #6560, #12086, .T. ) ;
#12637=ORIENTED_EDGE ( 'NONE', *, *, #21667, .T. ) ;
#12638=CARTESIAN_POINT ( 'NONE',  ( 39.31606138205700063, 43.19123852234599781, 74.30501292736987295 ) ) ;
#12645=CIRCLE ( 'NONE', #9772, 1.000000000000000888 ) ;
#12646=AXIS2_PLACEMENT_3D ( 'NONE', #24094, #8667, #10849 ) ;
#12655=LINE ( 'NONE', #6710, #18905 ) ;
#12664=ORIENTED_EDGE ( 'NONE', *, *, #14290, .T. ) ;
#12665=DIRECTION ( 'NONE',  ( 1.000000000000000000, 0.000000000000000000, 0.000000000000000000 ) ) ;
#12666=DIRECTION ( 'NONE',  ( 1.000000000000000000, 0.000000000000000000, 0.000000000000000000 ) ) ;
#12669=ORIENTED_EDGE ( 'NONE', *, *, #2690, .F. ) ;
#12676=DIRECTION ( 'NONE',  ( -1.000000000000000000, 5.204170427930413997E-31, 1.734723475976804876E-16 ) ) ;
#12677=CARTESIAN_POINT ( 'NONE',  ( 44.81606138205700063, -34.55876147765400930, 73.30501292737011454 ) ) ;
#12697=DIRECTION ( 'NONE',  ( 1.000000000000000000, 0.000000000000000000, 0.000000000000000000 ) ) ;
#12711=ORIENTED_EDGE ( 'NONE', *, *, #21435, .T. ) ;
#12712=LINE ( 'NONE', #24779, #13695 ) ;
#12728=DIRECTION ( 'NONE',  ( 1.000000000000000000, -1.115179377413661005E-30, -3.717264591378870232E-16 ) ) ;
#12733=ORIENTED_EDGE ( 'NONE', *, *, #2194, .F. ) ;
#12743=CIRCLE ( 'NONE', #3242, 2.499999999999998668 ) ;
#12754=AXIS2_PLACEMENT_3D ( 'NONE', #11333, #3192, #1003 ) ;
#12766=DIRECTION ( 'NONE',  ( 0.000000000000000000, 0.000000000000000000, 1.000000000000000000 ) ) ;
#12771=ORIENTED_EDGE ( 'NONE', *, *, #12959, .F. ) ;
#12777=AXIS2_PLACEMENT_3D ( 'NONE', #1665, #7486, #7749 ) ;
#12778=LINE ( 'NONE', #24333, #15168 ) ;
#12790=ORIENTED_EDGE ( 'NONE', *, *, #22005, .F. ) ;
#12791=CARTESIAN_POINT ( 'NONE',  ( 32.81606138205700773, -24.55876147765401285, 70.30501292737008612 ) ) ;
#12793=DIRECTION ( 'NONE',  ( -9.027796614315171564E-31, -1.000000000000000000, -3.938893903907230117E-15 ) ) ;
#12795=ORIENTED_EDGE ( 'NONE', *, *, #5924, .F. ) ;
#12796=CARTESIAN_POINT ( 'NONE',  ( 41.31606138205687273, 43.19123852234595518, 61.80501292736988006 ) ) ;
#12802=PLANE ( 'NONE',  #17217 ) ;
#12811=EDGE_CURVE ( 'NONE', #10286, #3155, #3027, .T. ) ;
#12813=VECTOR ( 'NONE', #23514, 1000.000000000000000 ) ;
#12825=VERTEX_POINT ( 'NONE', #24462 ) ;
#12839=AXIS2_PLACEMENT_3D ( 'NONE', #21943, #10608, #18091 ) ;
#12843=DIRECTION ( 'NONE',  ( 0.000000000000000000, 1.000000000000000000, -3.469446951953614189E-15 ) ) ;
#12853=ORIENTED_EDGE ( 'NONE', *, *, #1582, .F. ) ;
#12855=VECTOR ( 'NONE', #15150, 1000.000000000000000 ) ;
#12862=VERTEX_POINT ( 'NONE', #22422 ) ;
#12867=ADVANCED_FACE ( 'NONE', ( #8659 ), #2700, .F. ) ;
#12877=CARTESIAN_POINT ( 'NONE',  ( 40.81606138205700773, -31.05876147765399864, 74.30501292737010033 ) ) ;
#12889=VERTEX_POINT ( 'NONE', #15452 ) ;
#12890=CYLINDRICAL_SURFACE ( 'NONE', #19956, 1.000000000000000888 ) ;
#12895=CARTESIAN_POINT ( 'NONE',  ( 43.81606138205700063, 41.44123852234599070, 73.55501292736987295 ) ) ;
#12899=CIRCLE ( 'NONE', #14524, 1.000000000000000888 ) ;
#12908=FACE_OUTER_BOUND ( 'NONE', #11332, .T. ) ;
#12909=CIRCLE ( 'NONE', #3448, 1.000000000000000888 ) ;
#12910=ORIENTED_EDGE ( 'NONE', *, *, #1180, .F. ) ;
#12931=LINE ( 'NONE', #12677, #22130 ) ;
#12940=AXIS2_PLACEMENT_3D ( 'NONE', #12421, #16260, #14219 ) ;
#12948=CARTESIAN_POINT ( 'NONE',  ( 31.81606138205700418, -36.10876147765401356, 70.30501292737011454 ) ) ;
#12959=EDGE_CURVE ( 'NONE', #15432, #14470, #9300, .T. ) ;
#12964=ORIENTED_EDGE ( 'NONE', *, *, #1215, .T. ) ;
#12973=CYLINDRICAL_SURFACE ( 'NONE', #20928, 1.750000000000001554 ) ;
#12976=LINE ( 'NONE', #20824, #15203 ) ;
#12981=EDGE_LOOP ( 'NONE', ( #17358, #4029, #13723, #14391, #11497, #2910, #22080, #7434, #3915, #5309, #20836, #10173 ) ) ;
#12982=VECTOR ( 'NONE', #23704, 1000.000000000000000 ) ;
#12995=DIRECTION ( 'NONE',  ( 0.000000000000000000, -0.8213699656732942334, 0.5703958094953462954 ) ) ;
#13003=CYLINDRICAL_SURFACE ( 'NONE', #12754, 1.000000000000000888 ) ;
#13011=VERTEX_POINT ( 'NONE', #11477 ) ;
#13017=FACE_BOUND ( 'NONE', #12577, .T. ) ;
#13028=FACE_OUTER_BOUND ( 'NONE', #15784, .T. ) ;
#13029=VERTEX_POINT ( 'NONE', #18948 ) ;
#13031=DIRECTION ( 'NONE',  ( -9.027796614315171564E-31, -1.000000000000000000, -1.163336342344335610E-15 ) ) ;
#13046=EDGE_CURVE ( 'NONE', #8243, #4589, #11703, .T. ) ;
#13052=DIRECTION ( 'NONE',  ( 9.251858538542962756E-15, 1.000000000000000000, 0.000000000000000000 ) ) ;
#13053=VERTEX_POINT ( 'NONE', #21510 ) ;
#13077=LINE ( 'NONE', #3270, #2641 ) ;
#13079=ORIENTED_EDGE ( 'NONE', *, *, #24272, .T. ) ;
#13082=CIRCLE ( 'NONE', #19652, 1.000000000000000888 ) ;
#13084=LINE ( 'NONE', #13833, #1813 ) ;
#13093=ORIENTED_EDGE ( 'NONE', *, *, #1022, .T. ) ;
#13100=DIRECTION ( 'NONE',  ( -4.256992727861094749E-32, 1.000000000000000000, -3.115648231731786715E-15 ) ) ;
#13114=DIRECTION ( 'NONE',  ( 1.734723475976804876E-16, 2.999999999999999839E-15, 1.000000000000000000 ) ) ;
#13129=ADVANCED_FACE ( 'NONE', ( #10170 ), #18037, .F. ) ;
#13139=VECTOR ( 'NONE', #6180, 1000.000000000000000 ) ;
#13145=VERTEX_POINT ( 'NONE', #9796 ) ;
#13154=AXIS2_PLACEMENT_3D ( 'NONE', #4856, #3169, #24917 ) ;
#13165=VERTEX_POINT ( 'NONE', #17783 ) ;
#13174=DIRECTION ( 'NONE',  ( -1.000000000000000000, 0.000000000000000000, 0.000000000000000000 ) ) ;
#13202=LINE ( 'NONE', #12948, #23016 ) ;
#13208=CARTESIAN_POINT ( 'NONE',  ( 31.81606138205700418, 38.19123852234598360, 71.05501292736988717 ) ) ;
#13210=ORIENTED_EDGE ( 'NONE', *, *, #3112, .F. ) ;
#13221=VECTOR ( 'NONE', #18931, 1000.000000000000000 ) ;
#13225=( LENGTH_UNIT ( ) NAMED_UNIT ( * ) SI_UNIT ( .MILLI., .METRE. ) );
#13237=CARTESIAN_POINT ( 'NONE',  ( 32.81606138205700773, 28.12806996228107437, 66.30501292736992980 ) ) ;
#13248=AXIS2_PLACEMENT_3D ( 'NONE', #4525, #4647, #16237 ) ;
#13250=EDGE_CURVE ( 'NONE', #16702, #1954, #1230, .T. ) ;
#13262=VERTEX_POINT ( 'NONE', #5114 ) ;
#13264=CARTESIAN_POINT ( 'NONE',  ( 44.81606138205700063, 38.19123852234599070, 73.05501292736988717 ) ) ;
#13268=DIRECTION ( 'NONE',  ( 0.000000000000000000, 2.999999999999999839E-15, 1.000000000000000000 ) ) ;
#13273=FACE_OUTER_BOUND ( 'NONE', #24423, .T. ) ;
#13286=DIRECTION ( 'NONE',  ( 1.000000000000000000, 0.000000000000000000, 0.000000000000000000 ) ) ;
#13289=ORIENTED_EDGE ( 'NONE', *, *, #8085, .F. ) ;
#13291=VECTOR ( 'NONE', #21580, 1000.000000000000000 ) ;
#13297=LINE ( 'NONE', #7361, #13599 ) ;
#13302=CARTESIAN_POINT ( 'NONE',  ( 31.81606138205700418, -34.55876147765401640, 70.30501292737011454 ) ) ;
#13309=CIRCLE ( 'NONE', #22340, 1.000000000000000888 ) ;
#13311=VERTEX_POINT ( 'NONE', #968 ) ;
#13313=CIRCLE ( 'NONE', #22370, 1.000000000000000888 ) ;
#13325=VERTEX_POINT ( 'NONE', #24662 ) ;
#13342=DIRECTION ( 'NONE',  ( 0.000000000000000000, 2.999999999999999839E-15, 1.000000000000000000 ) ) ;
#13345=ORIENTED_EDGE ( 'NONE', *, *, #24011, .T. ) ;
#13346=CARTESIAN_POINT ( 'NONE',  ( 43.06606138205700063, 41.44123852234595518, 61.30501292736988006 ) ) ;
#13348=DIRECTION ( 'NONE',  ( -3.373073425510455500E-16, -2.999999999999999839E-15, -1.000000000000000000 ) ) ;
#13360=ORIENTED_EDGE ( 'NONE', *, *, #1531, .T. ) ;
#13361=VERTEX_POINT ( 'NONE', #22447 ) ;
#13364=DIRECTION ( 'NONE',  ( 1.000000000000000000, 0.000000000000000000, 0.000000000000000000 ) ) ;
#13370=DIRECTION ( 'NONE',  ( -1.000000000000000000, 5.510910596163088391E-31, 1.836970198721029688E-16 ) ) ;
#13372=EDGE_CURVE ( 'NONE', #21491, #1363, #987, .T. ) ;
#13379=EDGE_CURVE ( 'NONE', #9429, #20085, #3951, .T. ) ;
#13383=DIRECTION ( 'NONE',  ( -1.000000000000000000, 1.040834085586084551E-30, 3.469446951953615175E-16 ) ) ;
#13388=CARTESIAN_POINT ( 'NONE',  ( 44.81606138205700063, 38.19123852234598360, 71.05501292736988717 ) ) ;
#13391=VERTEX_POINT ( 'NONE', #201 ) ;
#13402=PLANE ( 'NONE',  #22738 ) ;
#13410=VERTEX_POINT ( 'NONE', #14591 ) ;
#13412=EDGE_CURVE ( 'NONE', #10709, #19565, #665, .T. ) ;
#13420=DIRECTION ( 'NONE',  ( 3.717264591378870232E-16, 3.130104260698260371E-15, 1.000000000000000000 ) ) ;
#13446=DIRECTION ( 'NONE',  ( -1.836970198721029688E-16, -2.999999999999999839E-15, -1.000000000000000000 ) ) ;
#13448=EDGE_LOOP ( 'NONE', ( #19558, #2676, #8539, #23816 ) ) ;
#13451=FACE_OUTER_BOUND ( 'NONE', #17973, .T. ) ;
#13463=DIRECTION ( 'NONE',  ( -1.836970198721029688E-16, -2.999999999999999839E-15, -1.000000000000000000 ) ) ;
#13466=CARTESIAN_POINT ( 'NONE',  ( 32.81606138205700773, -34.55876147765401640, 70.30501292737011454 ) ) ;
#13479=VECTOR ( 'NONE', #11, 1000.000000000000000 ) ;
#13480=AXIS2_PLACEMENT_3D ( 'NONE', #5614, #3674, #11558 ) ;
#13483=VERTEX_POINT ( 'NONE', #23519 ) ;
#13486=VERTEX_POINT ( 'NONE', #14468 ) ;
#13487=DIRECTION ( 'NONE',  ( -1.000000000000000000, 0.000000000000000000, 0.000000000000000000 ) ) ;
#13504=EDGE_LOOP ( 'NONE', ( #3551, #22557, #4660, #16905 ) ) ;
#13512=CARTESIAN_POINT ( 'NONE',  ( 44.81606138205700063, -24.55876147765401285, 70.30501292737008612 ) ) ;
#13522=( NAMED_UNIT ( * ) SI_UNIT ( $, .STERADIAN. ) SOLID_ANGLE_UNIT ( ) );
#13532=DIRECTION ( 'NONE',  ( 0.000000000000000000, 2.775557561562888984E-15, 1.000000000000000000 ) ) ;
#13537=VECTOR ( 'NONE', #3594, 1000.000000000000000 ) ;
#13550=CIRCLE ( 'NONE', #23411, 0.5000000000000004441 ) ;
#13557=ADVANCED_FACE ( 'NONE', ( #14362 ), #22086, .F. ) ;
#13559=ADVANCED_FACE ( 'NONE', ( #4194 ), #18359, .T. ) ;
#13564=AXIS2_PLACEMENT_3D ( 'NONE', #19825, #24301, #20206 ) ;
#13572=ORIENTED_EDGE ( 'NONE', *, *, #2699, .F. ) ;
#13576=CIRCLE ( 'NONE', #14402, 1.750000000000001554 ) ;
#13586=VECTOR ( 'NONE', #17934, 1000.000000000000000 ) ;
#13587=FACE_OUTER_BOUND ( 'NONE', #24274, .T. ) ;
#13589=ADVANCED_FACE ( 'NONE', ( #14113 ), #22346, .T. ) ;
#13590=ORIENTED_EDGE ( 'NONE', *, *, #5799, .T. ) ;
#13594=FACE_OUTER_BOUND ( 'NONE', #3672, .T. ) ;
#13598=ORIENTED_EDGE ( 'NONE', *, *, #3317, .F. ) ;
#13599=VECTOR ( 'NONE', #15464, 1000.000000000000000 ) ;
#13608=ORIENTED_EDGE ( 'NONE', *, *, #1022, .F. ) ;
#13620=DIRECTION ( 'NONE',  ( 0.000000000000000000, 6.938893903907222067E-15, 1.000000000000000000 ) ) ;
#13631=CARTESIAN_POINT ( 'NONE',  ( 40.31606138205700773, 37.94123852234599781, 74.30501292736988717 ) ) ;
#13642=ORIENTED_EDGE ( 'NONE', *, *, #18681, .T. ) ;
#13643=LINE ( 'NONE', #11727, #3080 ) ;
#13670=AXIS2_PLACEMENT_3D ( 'NONE', #16198, #22507, #4489 ) ;
#13684=EDGE_CURVE ( 'NONE', #17867, #2806, #2628, .T. ) ;
#13685=ADVANCED_FACE ( 'NONE', ( #4330 ), #12194, .F. ) ;
#13686=DIRECTION ( 'NONE',  ( 0.000000000000000000, 1.000000000000000000, -2.999999999999999839E-15 ) ) ;
#13695=VECTOR ( 'NONE', #9107, 1000.000000000000000 ) ;
#13701=CARTESIAN_POINT ( 'NONE',  ( 31.81606138205700418, -36.10876147765401356, 70.30501292737011454 ) ) ;
#13709=CIRCLE ( 'NONE', #14531, 0.5000000000000004441 ) ;
#13715=LINE ( 'NONE', #40, #19672 ) ;
#13719=LINE ( 'NONE', #7925, #20045 ) ;
#13722=LINE ( 'NONE', #17588, #13291 ) ;
#13723=ORIENTED_EDGE ( 'NONE', *, *, #16632, .T. ) ;
#13732=ORIENTED_EDGE ( 'NONE', *, *, #4712, .T. ) ;
#13733=VERTEX_POINT ( 'NONE', #14859 ) ;
#13737=ADVANCED_FACE ( 'NONE', ( #3265 ), #22849, .F. ) ;
#13741=EDGE_CURVE ( 'NONE', #8063, #12188, #18602, .T. ) ;
#13743=CARTESIAN_POINT ( 'NONE',  ( 43.06606138205700063, -34.55876147765400219, 74.30501292737011454 ) ) ;
#13751=ORIENTED_EDGE ( 'NONE', *, *, #16846, .F. ) ;
#13753=ORIENTED_EDGE ( 'NONE', *, *, #25099, .F. ) ;
#13763=ORIENTED_EDGE ( 'NONE', *, *, #1215, .F. ) ;
#13770=ORIENTED_EDGE ( 'NONE', *, *, #13988, .T. ) ;
#13771=DIRECTION ( 'NONE',  ( 0.000000000000000000, 1.000000000000000000, 0.000000000000000000 ) ) ;
#13781=AXIS2_PLACEMENT_3D ( 'NONE', #17801, #23451, #5818 ) ;
#13783=DIRECTION ( 'NONE',  ( 0.000000000000000000, -2.999999999999999839E-15, -1.000000000000000000 ) ) ;
#13790=EDGE_LOOP ( 'NONE', ( #14898, #25278, #1268, #15306 ) ) ;
#13797=DIRECTION ( 'NONE',  ( -1.000000000000000000, 7.144651197284802049E-31, 8.673617379884039170E-17 ) ) ;
#13805=DIRECTION ( 'NONE',  ( -1.000000000000000000, 5.510910596163088391E-31, 1.836970198721029688E-16 ) ) ;
#13808=CARTESIAN_POINT ( 'NONE',  ( 40.31606138205700773, 39.69123852234597649, 69.30501292736988717 ) ) ;
#13816=EDGE_CURVE ( 'NONE', #16707, #11368, #18649, .T. ) ;
#13827=EDGE_LOOP ( 'NONE', ( #8193, #18370, #5081, #9891 ) ) ;
#13828=ORIENTED_EDGE ( 'NONE', *, *, #13684, .T. ) ;
#13829=CARTESIAN_POINT ( 'NONE',  ( 31.81606138205700418, 35.95440708241085304, 62.30501292736990138 ) ) ;
#13833=CARTESIAN_POINT ( 'NONE',  ( 40.81606138205700773, 37.44123852234599781, 75.30501292736990138 ) ) ;
#13837=DIRECTION ( 'NONE',  ( -4.789116818843729608E-32, 1.000000000000000000, -3.130104260698260371E-15 ) ) ;
#13839=EDGE_LOOP ( 'NONE', ( #3470, #6058, #8041, #18129 ) ) ;
#13844=SURFACE_STYLE_USAGE ( .BOTH. , #15894 ) ;
#13845=FACE_OUTER_BOUND ( 'NONE', #13839, .T. ) ;
#13860=ORIENTED_EDGE ( 'NONE', *, *, #18715, .F. ) ;
#13861=ORIENTED_EDGE ( 'NONE', *, *, #3254, .F. ) ;
#13869=VECTOR ( 'NONE', #936, 1000.000000000000000 ) ;
#13874=VERTEX_POINT ( 'NONE', #13701 ) ;
#13879=EDGE_CURVE ( 'NONE', #20215, #7904, #7908, .T. ) ;
#13892=ORIENTED_EDGE ( 'NONE', *, *, #13816, .T. ) ;
#13899=SURFACE_STYLE_USAGE ( .BOTH. , #1902 ) ;
#13901=VECTOR ( 'NONE', #5895, 1000.000000000000000 ) ;
#13903=EDGE_CURVE ( 'NONE', #21773, #4055, #3422, .T. ) ;
#13907=LINE ( 'NONE', #4497, #23819 ) ;
#13908=DIRECTION ( 'NONE',  ( 1.000000000000000000, 0.000000000000000000, 0.000000000000000000 ) ) ;
#13909=LINE ( 'NONE', #741, #11919 ) ;
#13914=ORIENTED_EDGE ( 'NONE', *, *, #20700, .F. ) ;
#13918=CIRCLE ( 'NONE', #2792, 0.7500000000000006661 ) ;
#13920=EDGE_CURVE ( 'NONE', #19274, #20085, #5972, .T. ) ;
#13954=ORIENTED_EDGE ( 'NONE', *, *, #10837, .F. ) ;
#13965=EDGE_CURVE ( 'NONE', #4719, #13410, #25395, .T. ) ;
#13968=EDGE_CURVE ( 'NONE', #2309, #5235, #14929, .T. ) ;
#13969=DIRECTION ( 'NONE',  ( 0.000000000000000000, 2.775557561562888984E-15, 1.000000000000000000 ) ) ;
#13972=DIRECTION ( 'NONE',  ( 1.000000000000000000, 0.000000000000000000, 0.000000000000000000 ) ) ;
#13977=CARTESIAN_POINT ( 'NONE',  ( 31.81606138205700418, -38.55876147765400219, 75.30501292737012875 ) ) ;
#13984=EDGE_CURVE ( 'NONE', #4055, #21773, #13309, .T. ) ;
#13988=EDGE_CURVE ( 'NONE', #13325, #9870, #1461, .T. ) ;
#13995=CARTESIAN_POINT ( 'NONE',  ( 40.31606138205697221, 33.19123852234596939, 66.30501292736991559 ) ) ;
#14002=DIRECTION ( 'NONE',  ( 0.000000000000000000, 0.000000000000000000, -1.000000000000000000 ) ) ;
#14010=CARTESIAN_POINT ( 'NONE',  ( 38.31606138205700063, 39.69123852234598360, 71.30501292737018559 ) ) ;
#14017=CARTESIAN_POINT ( 'NONE',  ( 43.81606138205700063, 41.44123852234596939, 66.30501292736988717 ) ) ;
#14023=ORIENTED_EDGE ( 'NONE', *, *, #23804, .T. ) ;
#14026=AXIS2_PLACEMENT_3D ( 'NONE', #4259, #2301, #18042 ) ;
#14032=CARTESIAN_POINT ( 'NONE',  ( 31.81606138205700418, 41.44123852234599070, 73.55501292736987295 ) ) ;
#14038=DIRECTION ( 'NONE',  ( -1.000000000000000000, 0.000000000000000000, 0.000000000000000000 ) ) ;
#14042=PLANE ( 'NONE',  #14026 ) ;
#14048=PLANE ( 'NONE',  #10323 ) ;
#14070=DIRECTION ( 'NONE',  ( 0.000000000000000000, 3.469446951953611033E-15, 1.000000000000000000 ) ) ;
#14079=ORIENTED_EDGE ( 'NONE', *, *, #11311, .F. ) ;
#14108=DIRECTION ( 'NONE',  ( -1.000000000000000000, 1.115179377413661005E-30, 3.717264591378870232E-16 ) ) ;
#14112=VECTOR ( 'NONE', #17884, 1000.000000000000000 ) ;
#14113=FACE_OUTER_BOUND ( 'NONE', #8473, .T. ) ;
#14128=AXIS2_PLACEMENT_3D ( 'NONE', #18621, #16553, #1086 ) ;
#14129=CARTESIAN_POINT ( 'NONE',  ( 40.31606138205700773, 38.69123852234599070, 73.55501292736988717 ) ) ;
#14131=VERTEX_POINT ( 'NONE', #24101 ) ;
#14135=EDGE_CURVE ( 'NONE', #22793, #25358, #13709, .T. ) ;
#14137=AXIS2_PLACEMENT_3D ( 'NONE', #20150, #2485, #297 ) ;
#14138=LINE ( 'NONE', #15927, #14112 ) ;
#14139=CARTESIAN_POINT ( 'NONE',  ( 32.81606138205700773, 28.69846577177642288, 66.12638289304319983 ) ) ;
#14177=VECTOR ( 'NONE', #8681, 1000.000000000000000 ) ;
#14185=DIRECTION ( 'NONE',  ( -9.027796614315171564E-31, -1.000000000000000000, -3.938893903907230117E-15 ) ) ;
#14190=VECTOR ( 'NONE', #11369, 1000.000000000000000 ) ;
#14191=FACE_OUTER_BOUND ( 'NONE', #2661, .T. ) ;
#14206=AXIS2_PLACEMENT_3D ( 'NONE', #3467, #3845, #23289 ) ;
#14219=DIRECTION ( 'NONE',  ( 3.373073425510455500E-16, 2.999999999999999839E-15, 1.000000000000000000 ) ) ;
#14220=ADVANCED_FACE ( 'NONE', ( #2840 ), #16998, .F. ) ;
#14226=VERTEX_POINT ( 'NONE', #16504 ) ;
#14227=DIRECTION ( 'NONE',  ( 1.000000000000000000, -9.027796614315171564E-31, -4.436993566807132493E-46 ) ) ;
#14228=CARTESIAN_POINT ( 'NONE',  ( 44.81606138205700063, 35.95440708241085304, 61.30501292736990138 ) ) ;
#14234=DIRECTION ( 'NONE',  ( -1.000000000000000000, 0.000000000000000000, 0.000000000000000000 ) ) ;
#14236=DIRECTION ( 'NONE',  ( -3.373073425510455500E-16, -2.999999999999999839E-15, -1.000000000000000000 ) ) ;
#14240=ORIENTED_EDGE ( 'NONE', *, *, #10827, .F. ) ;
#14241=FACE_OUTER_BOUND ( 'NONE', #9397, .T. ) ;
#14256=VERTEX_POINT ( 'NONE', #13264 ) ;
#14257=ORIENTED_EDGE ( 'NONE', *, *, #14290, .F. ) ;
#14260=CARTESIAN_POINT ( 'NONE',  ( 40.31606138205700773, 37.94123852234599781, 74.30501292736988717 ) ) ;
#14264=CARTESIAN_POINT ( 'NONE',  ( 35.81606138205700063, 37.44123852234599781, 75.30501292736990138 ) ) ;
#14265=DIRECTION ( 'NONE',  ( 0.000000000000000000, 1.000000000000000000, -2.999999999999999839E-15 ) ) ;
#14271=ORIENTED_EDGE ( 'NONE', *, *, #19884, .F. ) ;
#14272=EDGE_CURVE ( 'NONE', #19241, #5247, #9284, .T. ) ;
#14290=EDGE_CURVE ( 'NONE', #1954, #8849, #14579, .T. ) ;
#14307=LINE ( 'NONE', #12257, #950 ) ;
#14309=CARTESIAN_POINT ( 'NONE',  ( 42.06606138205700063, 43.19123852234599781, 75.30501292736987295 ) ) ;
#14315=CYLINDRICAL_SURFACE ( 'NONE', #17177, 1.000000000000000888 ) ;
#14320=VECTOR ( 'NONE', #3241, 1000.000000000000000 ) ;
#14323=DIRECTION ( 'NONE',  ( 0.000000000000000000, 1.000000000000000000, -2.999999999999998655E-15 ) ) ;
#14340=ADVANCED_FACE ( 'NONE', ( #3579 ), #1636, .F. ) ;
#14342=ADVANCED_FACE ( 'NONE', ( #25335 ), #17767, .F. ) ;
#14343=MECHANICAL_DESIGN_GEOMETRIC_PRESENTATION_REPRESENTATION('',(#9829),#5698);
#14346=LINE ( 'NONE', #22199, #19070 ) ;
#14357=EDGE_LOOP ( 'NONE', ( #13210, #9344, #22144, #6297 ) ) ;
#14362=FACE_OUTER_BOUND ( 'NONE', #15995, .T. ) ;
#14369=DIRECTION ( 'NONE',  ( 0.000000000000000000, 2.775557561562888984E-15, 1.000000000000000000 ) ) ;
#14373=VECTOR ( 'NONE', #10687, 1000.000000000000000 ) ;
#14374=EDGE_CURVE ( 'NONE', #13145, #13325, #6164, .T. ) ;
#14384=VECTOR ( 'NONE', #6251, 1000.000000000000000 ) ;
#14389=FACE_OUTER_BOUND ( 'NONE', #18951, .T. ) ;
#14391=ORIENTED_EDGE ( 'NONE', *, *, #11635, .F. ) ;
#14395=AXIS2_PLACEMENT_3D ( 'NONE', #2804, #16217, #24068 ) ;
#14402=AXIS2_PLACEMENT_3D ( 'NONE', #5241, #20961, #7301 ) ;
#14404=CARTESIAN_POINT ( 'NONE',  ( 43.81606138205700063, 35.38401127291550097, 61.48364296169660292 ) ) ;
#14406=CIRCLE ( 'NONE', #16870, 4.000000000000000000 ) ;
#14408=DIRECTION ( 'NONE',  ( 1.000000000000000000, 0.000000000000000000, 0.000000000000000000 ) ) ;
#14412=APPLICATION_CONTEXT ( 'automotive_design' ) ;
#14414=ADVANCED_FACE ( 'NONE', ( #7980 ), #11723, .F. ) ;
#14420=VERTEX_POINT ( 'NONE', #23413 ) ;
#14421=ORIENTED_EDGE ( 'NONE', *, *, #7716, .T. ) ;
#14435=DIRECTION ( 'NONE',  ( 9.027796614315171564E-31, 1.000000000000000000, 1.163336342344335610E-15 ) ) ;
#14442=CARTESIAN_POINT ( 'NONE',  ( 40.31606138205700773, 42.19123852234596939, 65.30501292736988717 ) ) ;
#14444=DIRECTION ( 'NONE',  ( 0.000000000000000000, -1.000000000000000000, 3.325260651745651169E-15 ) ) ;
#14454=ORIENTED_EDGE ( 'NONE', *, *, #1528, .F. ) ;
#14459=ORIENTED_EDGE ( 'NONE', *, *, #6042, .F. ) ;
#14465=EDGE_CURVE ( 'NONE', #21608, #13262, #21880, .T. ) ;
#14468=CARTESIAN_POINT ( 'NONE',  ( 36.31606138205700063, 39.69123852234599070, 73.55501292736988717 ) ) ;
#14470=VERTEX_POINT ( 'NONE', #2030 ) ;
#14479=LINE ( 'NONE', #24120, #21815 ) ;
#14485=ORIENTED_EDGE ( 'NONE', *, *, #2320, .F. ) ;
#14487=CYLINDRICAL_SURFACE ( 'NONE', #5340, 2.000000000000001776 ) ;
#14492=EDGE_LOOP ( 'NONE', ( #14897, #14023, #18744, #4192 ) ) ;
#14504=ORIENTED_EDGE ( 'NONE', *, *, #94, .F. ) ;
#14505=CARTESIAN_POINT ( 'NONE',  ( 43.81606138205700063, 35.38401127291550097, 61.48364296169660292 ) ) ;
#14512=ADVANCED_FACE ( 'NONE', ( #2158 ), #10035, .F. ) ;
#14520=LINE ( 'NONE', #10408, #22289 ) ;
#14524=AXIS2_PLACEMENT_3D ( 'NONE', #17359, #17111, #7828 ) ;
#14531=AXIS2_PLACEMENT_3D ( 'NONE', #8285, #12414, #22055 ) ;
#14533=AXIS2_PLACEMENT_3D ( 'NONE', #673, #6866, #18470 ) ;
#14536=AXIS2_PLACEMENT_3D ( 'NONE', #33, #7913, #21432 ) ;
#14564=CIRCLE ( 'NONE', #6338, 0.7500000000000006661 ) ;
#14565=CARTESIAN_POINT ( 'NONE',  ( 34.56606138205700773, 43.19123852234599781, 74.30501292736987295 ) ) ;
#14568=ORIENTED_EDGE ( 'NONE', *, *, #13379, .T. ) ;
#14570=VERTEX_POINT ( 'NONE', #473 ) ;
#14572=DIRECTION ( 'NONE',  ( 1.000000000000000000, 0.000000000000000000, 0.000000000000000000 ) ) ;
#14579=LINE ( 'NONE', #21238, #22707 ) ;
#14584=DIRECTION ( 'NONE',  ( -1.000000000000000000, 0.000000000000000000, 0.000000000000000000 ) ) ;
#14588=DIRECTION ( 'NONE',  ( 0.000000000000000000, -1.000000000000000000, 2.999999999999999839E-15 ) ) ;
#14591=CARTESIAN_POINT ( 'NONE',  ( 40.81606138205700773, 41.44123852234599781, 74.30501292736987295 ) ) ;
#14599=EDGE_CURVE ( 'NONE', #7272, #11199, #8733, .T. ) ;
#14610=ORIENTED_EDGE ( 'NONE', *, *, #7661, .T. ) ;
#14618=CARTESIAN_POINT ( 'NONE',  ( 35.31606138205687273, 43.19123852234595518, 61.80501292736988006 ) ) ;
#14625=CARTESIAN_POINT ( 'NONE',  ( 35.31606138205687273, 33.19123852234596939, 65.30501292736991559 ) ) ;
#14628=ORIENTED_EDGE ( 'NONE', *, *, #12289, .F. ) ;
#14653=CARTESIAN_POINT ( 'NONE',  ( 40.81606138205700773, -31.05876147765399864, 74.30501292737010033 ) ) ;
#14661=DIRECTION ( 'NONE',  ( 0.000000000000000000, 2.999999999999999839E-15, 1.000000000000000000 ) ) ;
#14678=EDGE_CURVE ( 'NONE', #22327, #1199, #880, .T. ) ;
#14689=ORIENTED_EDGE ( 'NONE', *, *, #13412, .T. ) ;
#14695=DIRECTION ( 'NONE',  ( 9.027796614315171564E-31, 1.000000000000000000, 3.938893903907230117E-15 ) ) ;
#14696=VECTOR ( 'NONE', #13686, 1000.000000000000000 ) ;
#14706=LINE ( 'NONE', #14968, #25262 ) ;
#14713=DIRECTION ( 'NONE',  ( 0.000000000000000000, 0.000000000000000000, -1.000000000000000000 ) ) ;
#14722=DIRECTION ( 'NONE',  ( -1.000000000000000000, 5.510910596163088391E-31, 1.836970198721029688E-16 ) ) ;
#14727=DIRECTION ( 'NONE',  ( -1.000000000000000000, 1.115179377413661005E-30, 3.717264591378870232E-16 ) ) ;
#14754=ADVANCED_FACE ( 'NONE', ( #25050 ), #24542, .T. ) ;
#14767=DIRECTION ( 'NONE',  ( 1.000000000000000000, 1.817449160981365809E-30, -1.734723475976805122E-15 ) ) ;
#14776=DIRECTION ( 'NONE',  ( 1.000000000000000000, -5.204170427930413121E-31, -1.734723475976804876E-16 ) ) ;
#14787=CARTESIAN_POINT ( 'NONE',  ( 41.31606138205687273, 43.19123852234596939, 65.30501292736988717 ) ) ;
#14793=VECTOR ( 'NONE', #12060, 1000.000000000000000 ) ;
#14796=DIRECTION ( 'NONE',  ( 1.000000000000000000, 0.000000000000000000, 0.000000000000000000 ) ) ;
#14798=ORIENTED_EDGE ( 'NONE', *, *, #5157, .F. ) ;
#14801=ADVANCED_FACE ( 'NONE', ( #15031 ), #6923, .T. ) ;
#14805=ORIENTED_EDGE ( 'NONE', *, *, #9282, .F. ) ;
#14806=CARTESIAN_POINT ( 'NONE',  ( 43.81606138205700063, 41.44123852234597649, 67.80501292736988717 ) ) ;
#14809=ORIENTED_EDGE ( 'NONE', *, *, #2407, .T. ) ;
#14813=DIRECTION ( 'NONE',  ( 0.000000000000000000, -1.387778780781454037E-14, 1.000000000000000000 ) ) ;
#14815=VECTOR ( 'NONE', #12665, 1000.000000000000000 ) ;
#14826=EDGE_CURVE ( 'NONE', #20085, #2367, #1246, .T. ) ;
#14830=ORIENTED_EDGE ( 'NONE', *, *, #141, .F. ) ;
#14835=ORIENTED_EDGE ( 'NONE', *, *, #1513, .F. ) ;
#14843=DIRECTION ( 'NONE',  ( -1.000000000000000000, 5.204170427930415223E-30, 1.734723475976805122E-15 ) ) ;
#14845=FACE_OUTER_BOUND ( 'NONE', #17343, .T. ) ;
#14851=PLANE ( 'NONE',  #1175 ) ;
#14859=CARTESIAN_POINT ( 'NONE',  ( 34.81606138205687273, 43.19123852234595518, 61.30501292736988006 ) ) ;
#14886=ADVANCED_FACE ( 'NONE', ( #16970 ), #15283, .T. ) ;
#14888=VECTOR ( 'NONE', #14588, 1000.000000000000000 ) ;
#14890=ORIENTED_EDGE ( 'NONE', *, *, #25099, .T. ) ;
#14891=ORIENTED_EDGE ( 'NONE', *, *, #14599, .T. ) ;
#14893=CARTESIAN_POINT ( 'NONE',  ( 43.81606138205700063, -34.55876147765400930, 73.55501292737011454 ) ) ;
#14897=ORIENTED_EDGE ( 'NONE', *, *, #6170, .F. ) ;
#14898=ORIENTED_EDGE ( 'NONE', *, *, #6032, .T. ) ;
#14911=CARTESIAN_POINT ( 'NONE',  ( 35.31606138205687273, 33.19123852234596939, 65.30501292736991559 ) ) ;
#14919=DIRECTION ( 'NONE',  ( 0.000000000000000000, -1.000000000000000000, 2.999999999999999839E-15 ) ) ;
#14920=AXIS2_PLACEMENT_3D ( 'NONE', #25346, #14408, #17906 ) ;
#14922=ORIENTED_EDGE ( 'NONE', *, *, #4836, .T. ) ;
#14929=CIRCLE ( 'NONE', #23566, 1.750000000000001554 ) ;
#14931=CARTESIAN_POINT ( 'NONE',  ( 44.81606138205700063, -34.55876147765400930, 73.30501292737011454 ) ) ;
#14937=EDGE_CURVE ( 'NONE', #5642, #22433, #9583, .T. ) ;
#14954=DIRECTION ( 'NONE',  ( -3.717264591378870232E-16, -2.999999999999999839E-15, -1.000000000000000000 ) ) ;
#14960=ORIENTED_EDGE ( 'NONE', *, *, #17941, .F. ) ;
#14968=CARTESIAN_POINT ( 'NONE',  ( 44.81606138205700063, 38.19123852234598360, 71.05501292736988717 ) ) ;
#14969=CARTESIAN_POINT ( 'NONE',  ( 35.31606138205687273, 33.19123852234596939, 65.30501292736991559 ) ) ;
#14976=VECTOR ( 'NONE', #4464, 1000.000000000000000 ) ;
#14979=VERTEX_POINT ( 'NONE', #5881 ) ;
#14980=EDGE_CURVE ( 'NONE', #13361, #9366, #8752, .T. ) ;
#14999=EDGE_LOOP ( 'NONE', ( #18148, #6778, #18998, #20861 ) ) ;
#15005=CARTESIAN_POINT ( 'NONE',  ( 43.06606138205700063, -34.55876147765400930, 73.55501292737011454 ) ) ;
#15008=EDGE_LOOP ( 'NONE', ( #4085, #53, #6730, #701 ) ) ;
#15014=CARTESIAN_POINT ( 'NONE',  ( 44.81606138205700063, 35.44123852234597649, 67.80501292736990138 ) ) ;
#15021=ADVANCED_FACE ( 'NONE', ( #19402 ), #21599, .F. ) ;
#15022=DIRECTION ( 'NONE',  ( 9.027796614315171564E-31, 1.000000000000000000, 1.163336342344335610E-15 ) ) ;
#15024=ORIENTED_EDGE ( 'NONE', *, *, #11980, .F. ) ;
#15029=ORIENTED_EDGE ( 'NONE', *, *, #11831, .F. ) ;
#15031=FACE_OUTER_BOUND ( 'NONE', #7664, .T. ) ;
#15044=FACE_OUTER_BOUND ( 'NONE', #20682, .T. ) ;
#15056=LINE ( 'NONE', #24451, #1016 ) ;
#15074=CARTESIAN_POINT ( 'NONE',  ( 44.81606138205700063, -24.55876147765401996, 67.80501292737008612 ) ) ;
#15087=AXIS2_PLACEMENT_3D ( 'NONE', #15264, #23631, #15773 ) ;
#15091=LINE ( 'NONE', #22945, #10089 ) ;
#15099=ORIENTED_EDGE ( 'NONE', *, *, #20191, .F. ) ;
#15100=PLANE ( 'NONE',  #24772 ) ;
#15108=CARTESIAN_POINT ( 'NONE',  ( 31.81606138205700418, 18.19123852234599426, 73.05501292736995822 ) ) ;
#15120=EDGE_CURVE ( 'NONE', #3155, #8442, #444, .T. ) ;
#15121=ORIENTED_EDGE ( 'NONE', *, *, #14465, .T. ) ;
#15124=ORIENTED_EDGE ( 'NONE', *, *, #3161, .T. ) ;
#15127=EDGE_CURVE ( 'NONE', #1199, #14256, #12327, .T. ) ;
#15141=AXIS2_PLACEMENT_3D ( 'NONE', #24040, #14265, #23788 ) ;
#15142=DIRECTION ( 'NONE',  ( -1.000000000000000000, 0.000000000000000000, 0.000000000000000000 ) ) ;
#15149=ORIENTED_EDGE ( 'NONE', *, *, #6875, .F. ) ;
#15150=DIRECTION ( 'NONE',  ( 3.028377322213060447E-31, 1.000000000000000000, -2.999999999999999839E-15 ) ) ;
#15167=CARTESIAN_POINT ( 'NONE',  ( 39.31606138205700063, 43.19123852234595518, 61.30501292736988006 ) ) ;
#15168=VECTOR ( 'NONE', #17015, 1000.000000000000000 ) ;
#15169=DIRECTION ( 'NONE',  ( 0.000000000000000000, 1.163336342344340343E-15, -1.000000000000000000 ) ) ;
#15172=CARTESIAN_POINT ( 'NONE',  ( 31.81606138205700418, -34.55876147765401640, 70.30501292737011454 ) ) ;
#15176=ORIENTED_EDGE ( 'NONE', *, *, #4836, .F. ) ;
#15183=DIRECTION ( 'NONE',  ( 0.000000000000000000, -1.000000000000000000, 2.999999999999999839E-15 ) ) ;
#15189=DIRECTION ( 'NONE',  ( 1.836970198721029688E-16, 2.999999999999999839E-15, 1.000000000000000000 ) ) ;
#15191=VECTOR ( 'NONE', #5290, 1000.000000000000000 ) ;
#15203=VECTOR ( 'NONE', #3159, 1000.000000000000000 ) ;
#15205=EDGE_CURVE ( 'NONE', #23679, #24313, #10805, .T. ) ;
#15213=EDGE_CURVE ( 'NONE', #13483, #16994, #10512, .T. ) ;
#15217=DIRECTION ( 'NONE',  ( -1.000000000000000000, 5.204170427930413997E-31, 1.734723475976804876E-16 ) ) ;
#15226=ORIENTED_EDGE ( 'NONE', *, *, #5176, .T. ) ;
#15238=EDGE_CURVE ( 'NONE', #4719, #9093, #24394, .T. ) ;
#15239=AXIS2_PLACEMENT_3D ( 'NONE', #4336, #4457, #20544 ) ;
#15244=CARTESIAN_POINT ( 'NONE',  ( 43.06606138205700063, 43.19123852234599070, 73.55501292736987295 ) ) ;
#15246=VECTOR ( 'NONE', #24559, 1000.000000000000000 ) ;
#15248=ADVANCED_FACE ( 'NONE', ( #8196, #8710, #16542, #12073 ), #9226, .F. ) ;
#15250=ORIENTED_EDGE ( 'NONE', *, *, #6905, .F. ) ;
#15259=DIRECTION ( 'NONE',  ( 1.000000000000000000, 0.000000000000000000, 0.000000000000000000 ) ) ;
#15262=CARTESIAN_POINT ( 'NONE',  ( 40.81606138205700773, 37.44123852234599781, 74.30501292736988717 ) ) ;
#15264=CARTESIAN_POINT ( 'NONE',  ( 44.81606138205700063, 35.95440708241085304, 62.30501292736990138 ) ) ;
#15265=LINE ( 'NONE', #24904, #21716 ) ;
#15272=LINE ( 'NONE', #9622, #15504 ) ;
#15283=PLANE ( 'NONE',  #7103 ) ;
#15289=ORIENTED_EDGE ( 'NONE', *, *, #10193, .T. ) ;
#15298=VECTOR ( 'NONE', #23898, 1000.000000000000000 ) ;
#15306=ORIENTED_EDGE ( 'NONE', *, *, #10967, .F. ) ;
#15314=FACE_OUTER_BOUND ( 'NONE', #7882, .T. ) ;
#15318=CARTESIAN_POINT ( 'NONE',  ( 43.81606138205700063, 41.44123852234595518, 61.30501292736988006 ) ) ;
#15321=AXIS2_PLACEMENT_3D ( 'NONE', #23771, #23383, #7818 ) ;
#15323=CIRCLE ( 'NONE', #5050, 1.000000000000000888 ) ;
#15329=DIRECTION ( 'NONE',  ( 1.117439894383781939E-44, -1.000000000000000000, 2.999999999999993528E-15 ) ) ;
#15332=ORIENTED_EDGE ( 'NONE', *, *, #19977, .T. ) ;
#15334=AXIS2_PLACEMENT_3D ( 'NONE', #14010, #707, #21863 ) ;
#15340=ORIENTED_EDGE ( 'NONE', *, *, #16478, .T. ) ;
#15341=DIRECTION ( 'NONE',  ( 1.836970198721029688E-16, 2.999999999999999839E-15, 1.000000000000000000 ) ) ;
#15351=FACE_OUTER_BOUND ( 'NONE', #7429, .T. ) ;
#15353=AXIS2_PLACEMENT_3D ( 'NONE', #20525, #4940, #24490 ) ;
#15360=CARTESIAN_POINT ( 'NONE',  ( 43.06606138205700063, 42.19123852234599781, 74.30501292736987295 ) ) ;
#15369=VERTEX_POINT ( 'NONE', #21059 ) ;
#15371=AXIS2_PLACEMENT_3D ( 'NONE', #355, #13783, #9924 ) ;
#15379=EDGE_LOOP ( 'NONE', ( #19646, #24391, #1084, #16945 ) ) ;
#15382=DIRECTION ( 'NONE',  ( -1.000000000000000000, 5.204170427930413997E-31, 1.734723475976804876E-16 ) ) ;
#15383=CARTESIAN_POINT ( 'NONE',  ( 31.81606138205700418, 41.44123852234595518, 61.30501292736988006 ) ) ;
#15394=VECTOR ( 'NONE', #12676, 1000.000000000000000 ) ;
#15399=ORIENTED_EDGE ( 'NONE', *, *, #3981, .T. ) ;
#15402=CARTESIAN_POINT ( 'NONE',  ( 36.31606138205700063, 39.69123852234597649, 69.30501292736988717 ) ) ;
#15407=DIRECTION ( 'NONE',  ( 0.000000000000000000, 0.000000000000000000, 1.000000000000000000 ) ) ;
#15431=DIRECTION ( 'NONE',  ( 5.642372883946980038E-32, 1.000000000000000000, -2.848211695852029218E-15 ) ) ;
#15432=VERTEX_POINT ( 'NONE', #23481 ) ;
#15434=ORIENTED_EDGE ( 'NONE', *, *, #11819, .T. ) ;
#15447=PRESENTATION_STYLE_ASSIGNMENT (( #13899 ) ) ;
#15449=DIRECTION ( 'NONE',  ( 0.000000000000000000, 1.000000000000000000, 0.000000000000000000 ) ) ;
#15452=CARTESIAN_POINT ( 'NONE',  ( 31.81606138205700418, -38.55876147765401640, 70.30501292737012875 ) ) ;
#15455=VERTEX_POINT ( 'NONE', #21186 ) ;
#15464=DIRECTION ( 'NONE',  ( 0.000000000000000000, -2.999999999999999839E-15, -1.000000000000000000 ) ) ;
#15501=DIRECTION ( 'NONE',  ( 1.000000000000000000, -6.938893903907219830E-30, -2.312964634635740294E-15 ) ) ;
#15503=LINE ( 'NONE', #11289, #22933 ) ;
#15504=VECTOR ( 'NONE', #5736, 1000.000000000000114 ) ;
#15506=ORIENTED_EDGE ( 'NONE', *, *, #20043, .T. ) ;
#15534=DIRECTION ( 'NONE',  ( -1.000000000000000000, 0.000000000000000000, 0.000000000000000000 ) ) ;
#15535=DIRECTION ( 'NONE',  ( 0.000000000000000000, -1.000000000000000000, 2.999999999999999839E-15 ) ) ;
#15537=ADVANCED_FACE ( 'NONE', ( #13451 ), #5845, .F. ) ;
#15553=CARTESIAN_POINT ( 'NONE',  ( 43.06606138205700063, 41.44123852234595518, 61.30501292736988006 ) ) ;
#15557=EDGE_LOOP ( 'NONE', ( #18990, #4074, #7959, #982 ) ) ;
#15558=CARTESIAN_POINT ( 'NONE',  ( 44.81606138205700063, 1.441238522345979600, 68.80501292737000085 ) ) ;
#15564=CARTESIAN_POINT ( 'NONE',  ( 43.06606138205700063, 41.44123852234599781, 75.30501292736987295 ) ) ;
#15573=DIRECTION ( 'NONE',  ( 1.000000000000000000, 0.000000000000000000, 0.000000000000000000 ) ) ;
#15584=EDGE_LOOP ( 'NONE', ( #8081, #24261 ) ) ;
#15592=AXIS2_PLACEMENT_3D ( 'NONE', #15172, #11452, #21108 ) ;
#15593=DIRECTION ( 'NONE',  ( -1.000000000000000000, 1.115179377413661005E-30, 3.717264591378870232E-16 ) ) ;
#15595=DIRECTION ( 'NONE',  ( 1.000000000000000000, -6.718359089036943783E-31, -1.734723475976804876E-16 ) ) ;
#15596=FACE_OUTER_BOUND ( 'NONE', #1036, .T. ) ;
#15604=VECTOR ( 'NONE', #20705, 1000.000000000000000 ) ;
#15613=VECTOR ( 'NONE', #8491, 1000.000000000000000 ) ;
#15623=DIRECTION ( 'NONE',  ( -1.000000000000000000, 5.630462536178272263E-31, 8.673617379884039170E-17 ) ) ;
#15624=DIRECTION ( 'NONE',  ( -1.000000000000000000, 1.115179377413661005E-30, 3.717264591378870232E-16 ) ) ;
#15628=VECTOR ( 'NONE', #6222, 1000.000000000000000 ) ;
#15637=LINE ( 'NONE', #1708, #18296 ) ;
#15643=CARTESIAN_POINT ( 'NONE',  ( 32.81606138205700773, 41.44123852234598360, 71.05501292736988717 ) ) ;
#15650=LINE ( 'NONE', #3541, #16433 ) ;
#15660=ORIENTED_EDGE ( 'NONE', *, *, #3487, .F. ) ;
#15661=VERTEX_POINT ( 'NONE', #6479 ) ;
#15683=DIRECTION ( 'NONE',  ( 0.000000000000000000, 2.999999999999999839E-15, 1.000000000000000000 ) ) ;
#15692=CARTESIAN_POINT ( 'NONE',  ( 40.81606138205700773, 37.44123852234599781, 75.30501292736990138 ) ) ;
#15709=EDGE_CURVE ( 'NONE', #13733, #8317, #23856, .T. ) ;
#15722=AXIS2_PLACEMENT_3D ( 'NONE', #23658, #15801, #8332 ) ;
#15726=VECTOR ( 'NONE', #15809, 1000.000000000000000 ) ;
#15731=LINE ( 'NONE', #7491, #17080 ) ;
#15732=DIRECTION ( 'NONE',  ( -1.000000000000000000, 0.000000000000000000, 0.000000000000000000 ) ) ;
#15773=DIRECTION ( 'NONE',  ( 0.000000000000000000, 1.000000000000000000, 0.000000000000000000 ) ) ;
#15776=ORIENTED_EDGE ( 'NONE', *, *, #10358, .T. ) ;
#15784=EDGE_LOOP ( 'NONE', ( #10569, #12584, #6845, #20785 ) ) ;
#15787=VERTEX_POINT ( 'NONE', #18711 ) ;
#15791=VERTEX_POINT ( 'NONE', #6987 ) ;
#15796=ORIENTED_EDGE ( 'NONE', *, *, #1119, .F. ) ;
#15801=DIRECTION ( 'NONE',  ( -1.000000000000000000, 1.040834085586084551E-30, 3.469446951953615175E-16 ) ) ;
#15809=DIRECTION ( 'NONE',  ( -1.000000000000000000, 1.115179377413661005E-30, 3.717264591378870232E-16 ) ) ;
#15812=ADVANCED_FACE ( 'NONE', ( #22946 ), #8925, .F. ) ;
#15818=ORIENTED_EDGE ( 'NONE', *, *, #19837, .T. ) ;
#15827=FILL_AREA_STYLE ('',( #7860 ) ) ;
#15831=CARTESIAN_POINT ( 'NONE',  ( 40.31606138205700773, -31.05876147765399864, 74.30501292737010033 ) ) ;
#15834=CARTESIAN_POINT ( 'NONE',  ( 32.81606138205700773, -38.55876147765401640, 70.30501292737012875 ) ) ;
#15840=ORIENTED_EDGE ( 'NONE', *, *, #5702, .T. ) ;
#15850=EDGE_LOOP ( 'NONE', ( #9744, #17185, #3539, #1419 ) ) ;
#15855=EDGE_CURVE ( 'NONE', #5247, #23734, #18246, .T. ) ;
#15884=DIRECTION ( 'NONE',  ( 0.000000000000000000, 0.000000000000000000, -1.000000000000000000 ) ) ;
#15888=VERTEX_POINT ( 'NONE', #16646 ) ;
#15891=FACE_OUTER_BOUND ( 'NONE', #23513, .T. ) ;
#15894=SURFACE_SIDE_STYLE ('',( #12304 ) ) ;
#15895=LINE ( 'NONE', #7930, #21920 ) ;
#15897=LINE ( 'NONE', #21582, #10675 ) ;
#15904=CARTESIAN_POINT ( 'NONE',  ( 43.81606138205700063, -22.55876147765401996, 68.80501292737008612 ) ) ;
#15907=CARTESIAN_POINT ( 'NONE',  ( 38.31606138205700063, 42.51966564709218233, 71.30501292737018559 ) ) ;
#15922=ORIENTED_EDGE ( 'NONE', *, *, #1840, .F. ) ;
#15927=CARTESIAN_POINT ( 'NONE',  ( 44.81606138205700063, -34.55876147765400219, 75.30501292737011454 ) ) ;
#15938=VERTEX_POINT ( 'NONE', #16511 ) ;
#15953=CARTESIAN_POINT ( 'NONE',  ( 36.31606138205700063, 37.94123852234599781, 75.30501292736988717 ) ) ;
#15957=ORIENTED_EDGE ( 'NONE', *, *, #717, .T. ) ;
#15972=EDGE_CURVE ( 'NONE', #16502, #10392, #12909, .T. ) ;
#15984=ADVANCED_FACE ( 'NONE', ( #7754 ), #1804, .T. ) ;
#15988=ADVANCED_FACE ( 'NONE', ( #15596 ), #5434, .T. ) ;
#15995=EDGE_LOOP ( 'NONE', ( #15176, #12795, #10038, #23761 ) ) ;
#15997=ORIENTED_EDGE ( 'NONE', *, *, #16488, .F. ) ;
#15998=LINE ( 'NONE', #23849, #14815 ) ;
#16013=VECTOR ( 'NONE', #595, 1000.000000000000000 ) ;
#16023=DIRECTION ( 'NONE',  ( -1.000000000000000000, 5.204170427930415223E-30, 1.734723475976805122E-15 ) ) ;
#16028=EDGE_CURVE ( 'NONE', #9377, #9429, #1672, .T. ) ;
#16033=ORIENTED_EDGE ( 'NONE', *, *, #16814, .T. ) ;
#16034=DIRECTION ( 'NONE',  ( -1.000000000000000000, 0.000000000000000000, 0.000000000000000000 ) ) ;
#16043=VERTEX_POINT ( 'NONE', #25246 ) ;
#16044=EDGE_CURVE ( 'NONE', #3140, #17954, #19464, .T. ) ;
#16064=CARTESIAN_POINT ( 'NONE',  ( 32.81606138205700773, 35.38401127291550097, 61.48364296169660292 ) ) ;
#16074=ORIENTED_EDGE ( 'NONE', *, *, #4100, .T. ) ;
#16083=LINE ( 'NONE', #4250, #12320 ) ;
#16088=ORIENTED_EDGE ( 'NONE', *, *, #5157, .T. ) ;
#16093=ORIENTED_EDGE ( 'NONE', *, *, #13412, .F. ) ;
#16102=EDGE_CURVE ( 'NONE', #5023, #25151, #17859, .T. ) ;
#16103=DIRECTION ( 'NONE',  ( 0.000000000000000000, 1.163336342344335610E-15, -1.000000000000000000 ) ) ;
#16118=VECTOR ( 'NONE', #19818, 1000.000000000000000 ) ;
#16120=CARTESIAN_POINT ( 'NONE',  ( 38.31606138205687273, 42.19123852234595518, 61.30501292736988006 ) ) ;
#16121=VECTOR ( 'NONE', #2902, 1000.000000000000000 ) ;
#16126=DIRECTION ( 'NONE',  ( 0.000000000000000000, 3.129456975819164530E-15, 1.000000000000000000 ) ) ;
#16129=ORIENTED_EDGE ( 'NONE', *, *, #10182, .T. ) ;
#16138=EDGE_LOOP ( 'NONE', ( #9718, #17448 ) ) ;
#16141=AXIS2_PLACEMENT_3D ( 'NONE', #17074, #20808, #22475 ) ;
#16144=FACE_OUTER_BOUND ( 'NONE', #17573, .T. ) ;
#16169=CARTESIAN_POINT ( 'NONE',  ( 36.31606138205700063, 39.69123852234597649, 69.30501292736988717 ) ) ;
#16177=EDGE_CURVE ( 'NONE', #16934, #7904, #13313, .T. ) ;
#16182=DIRECTION ( 'NONE',  ( -1.000000000000000000, 5.204170427930415223E-30, 1.734723475976805122E-15 ) ) ;
#16185=CARTESIAN_POINT ( 'NONE',  ( 43.81606138205700063, -36.55876147765400930, 73.30501292737011454 ) ) ;
#16191=PLANE ( 'NONE',  #15141 ) ;
#16193=ORIENTED_EDGE ( 'NONE', *, *, #22216, .T. ) ;
#16198=CARTESIAN_POINT ( 'NONE',  ( 40.31606138205700773, 43.19123852234599781, 74.30501292736987295 ) ) ;
#16206=DIRECTION ( 'NONE',  ( 1.000000000000000000, -3.982629455510873500E-31, -4.336808689942015271E-16 ) ) ;
#16212=VECTOR ( 'NONE', #24363, 1000.000000000000000 ) ;
#16217=DIRECTION ( 'NONE',  ( -0.000000000000000000, -1.000000000000000000, 2.999999999999998655E-15 ) ) ;
#16220=ORIENTED_EDGE ( 'NONE', *, *, #19959, .F. ) ;
#16237=DIRECTION ( 'NONE',  ( 0.000000000000000000, -3.469446951953611033E-15, -1.000000000000000000 ) ) ;
#16247=EDGE_CURVE ( 'NONE', #17440, #25304, #14307, .T. ) ;
#16252=ORIENTED_EDGE ( 'NONE', *, *, #24831, .F. ) ;
#16260=DIRECTION ( 'NONE',  ( -1.000000000000000000, 1.011922027653136605E-30, 3.373073425510455500E-16 ) ) ;
#16265=EDGE_CURVE ( 'NONE', #6560, #17850, #22154, .T. ) ;
#16268=ORIENTED_EDGE ( 'NONE', *, *, #10967, .T. ) ;
#16269=LINE ( 'NONE', #20650, #23171 ) ;
#16276=CARTESIAN_POINT ( 'NONE',  ( 40.31606138205700773, 37.44123852234599781, 74.30501292736988717 ) ) ;
#16279=ORIENTED_EDGE ( 'NONE', *, *, #23733, .F. ) ;
#16281=CARTESIAN_POINT ( 'NONE',  ( 44.81606138205700063, 35.44123852234597649, 68.30501292736990138 ) ) ;
#16289=ORIENTED_EDGE ( 'NONE', *, *, #15127, .F. ) ;
#16297=CARTESIAN_POINT ( 'NONE',  ( 44.81606138205700063, 38.19123852234599070, 72.05501292736988717 ) ) ;
#16320=FACE_OUTER_BOUND ( 'NONE', #9904, .T. ) ;
#16323=LINE ( 'NONE', #10042, #15613 ) ;
#16324=DIRECTION ( 'NONE',  ( 0.000000000000000000, 1.000000000000000000, -2.999999999999999839E-15 ) ) ;
#16339=EDGE_CURVE ( 'NONE', #17824, #4130, #18800, .T. ) ;
#16341=DIRECTION ( 'NONE',  ( 0.000000000000000000, 3.469446951953611033E-15, 1.000000000000000000 ) ) ;
#16347=VERTEX_POINT ( 'NONE', #2815 ) ;
#16355=PLANE ( 'NONE',  #20792 ) ;
#16359=AXIS2_PLACEMENT_3D ( 'NONE', #23578, #13797, #19716 ) ;
#16366=EDGE_LOOP ( 'NONE', ( #9370, #3911, #7859, #7723 ) ) ;
#16377=ORIENTED_EDGE ( 'NONE', *, *, #2541, .F. ) ;
#16382=DIRECTION ( 'NONE',  ( 0.000000000000000000, 1.000000000000000000, 0.000000000000000000 ) ) ;
#16403=AXIS2_PLACEMENT_3D ( 'NONE', #10876, #16789, #8694 ) ;
#16409=DIRECTION ( 'NONE',  ( 0.000000000000000000, -1.000000000000000000, 2.999999999999999839E-15 ) ) ;
#16411=AXIS2_PLACEMENT_3D ( 'NONE', #22895, #5261, #15169 ) ;
#16421=CARTESIAN_POINT ( 'NONE',  ( 36.31606138205700063, -31.05876147765399864, 74.30501292737010033 ) ) ;
#16429=LINE ( 'NONE', #24280, #18423 ) ;
#16430=DIRECTION ( 'NONE',  ( 1.000000000000000000, -5.204170427930415223E-30, -1.734723475976805122E-15 ) ) ;
#16432=CARTESIAN_POINT ( 'NONE',  ( 32.81606138205700773, 38.19123852234599070, 73.05501292736988717 ) ) ;
#16433=VECTOR ( 'NONE', #5607, 1000.000000000000000 ) ;
#16460=DIRECTION ( 'NONE',  ( -6.938893903907229955E-15, 1.000000000000000000, -2.999999999999999839E-15 ) ) ;
#16466=ORIENTED_EDGE ( 'NONE', *, *, #16339, .T. ) ;
#16470=FACE_OUTER_BOUND ( 'NONE', #19647, .T. ) ;
#16471=LINE ( 'NONE', #20608, #9386 ) ;
#16478=EDGE_CURVE ( 'NONE', #19565, #25152, #5406, .T. ) ;
#16480=LINE ( 'NONE', #16612, #23934 ) ;
#16486=ADVANCED_FACE ( 'NONE', ( #15314 ), #23419, .F. ) ;
#16488=EDGE_CURVE ( 'NONE', #22023, #15369, #16601, .T. ) ;
#16502=VERTEX_POINT ( 'NONE', #1406 ) ;
#16504=CARTESIAN_POINT ( 'NONE',  ( 43.81606138205700063, 41.44123852234595518, 61.30501292736988006 ) ) ;
#16510=DIRECTION ( 'NONE',  ( -1.000000000000000000, 5.510910596163088391E-31, 1.836970198721029688E-16 ) ) ;
#16511=CARTESIAN_POINT ( 'NONE',  ( 40.31606138205700773, -29.30876147765401640, 69.30501292737010033 ) ) ;
#16517=DIRECTION ( 'NONE',  ( -4.336808689942020201E-16, -2.999999999999999839E-15, -1.000000000000000000 ) ) ;
#16519=DIRECTION ( 'NONE',  ( 0.000000000000000000, -1.000000000000000000, 2.999999999999999839E-15 ) ) ;
#16526=AXIS2_PLACEMENT_3D ( 'NONE', #3209, #1019, #24711 ) ;
#16542=FACE_BOUND ( 'NONE', #18086, .T. ) ;
#16552=ORIENTED_EDGE ( 'NONE', *, *, #25340, .F. ) ;
#16553=DIRECTION ( 'NONE',  ( 1.836970198721029688E-16, 2.999999999999999839E-15, 1.000000000000000000 ) ) ;
#16558=CARTESIAN_POINT ( 'NONE',  ( 40.81606138205700773, -24.05876147765400219, 74.30501292737008612 ) ) ;
#16565=EDGE_LOOP ( 'NONE', ( #16938, #8064, #15957, #10882 ) ) ;
#16568=EDGE_CURVE ( 'NONE', #4444, #5522, #11728, .T. ) ;
#16571=EDGE_CURVE ( 'NONE', #13311, #5909, #21498, .T. ) ;
#16573=ORIENTED_EDGE ( 'NONE', *, *, #881, .F. ) ;
#16586=EDGE_CURVE ( 'NONE', #14226, #17824, #17516, .T. ) ;
#16588=LINE ( 'NONE', #22515, #11428 ) ;
#16596=DIRECTION ( 'NONE',  ( 1.734723475976804876E-16, -1.163336342344335610E-15, 1.000000000000000000 ) ) ;
#16601=CIRCLE ( 'NONE', #5931, 1.000000000000000888 ) ;
#16612=CARTESIAN_POINT ( 'NONE',  ( 41.31606138205687273, 43.19123852234595518, 61.30501292736988006 ) ) ;
#16619=AXIS2_PLACEMENT_3D ( 'NONE', #15907, #2371, #3003 ) ;
#16629=EDGE_CURVE ( 'NONE', #17824, #4719, #14564, .T. ) ;
#16632=EDGE_CURVE ( 'NONE', #18444, #10990, #19185, .T. ) ;
#16636=EDGE_LOOP ( 'NONE', ( #2662, #1907, #23390, #4102, #4815, #1129, #23224, #745, #10671, #1473, #5630, #5752 ) ) ;
#16646=CARTESIAN_POINT ( 'NONE',  ( 36.31606138205700063, 43.19123852234596939, 65.30501292736988717 ) ) ;
#16660=VECTOR ( 'NONE', #875, 1000.000000000000000 ) ;
#16668=ORIENTED_EDGE ( 'NONE', *, *, #11729, .T. ) ;
#16685=CARTESIAN_POINT ( 'NONE',  ( 40.31606138205700773, 43.19123852234596939, 66.30501292736988717 ) ) ;
#16692=DIRECTION ( 'NONE',  ( -3.491481338843135327E-15, -1.000000000000000000, 3.000000000000000628E-15 ) ) ;
#16695=DIRECTION ( 'NONE',  ( 0.000000000000000000, -2.999999999999999839E-15, -1.000000000000000000 ) ) ;
#16699=CARTESIAN_POINT ( 'NONE',  ( 40.31606138205700773, 37.44123852234599781, 75.30501292736990138 ) ) ;
#16700=CYLINDRICAL_SURFACE ( 'NONE', #6224, 0.7500000000000006661 ) ;
#16702=VERTEX_POINT ( 'NONE', #449 ) ;
#16707=VERTEX_POINT ( 'NONE', #16421 ) ;
#16708=ORIENTED_EDGE ( 'NONE', *, *, #11171, .F. ) ;
#16712=CARTESIAN_POINT ( 'NONE',  ( 33.56606138205700773, 43.19123852234599781, 74.30501292736987295 ) ) ;
#16715=LINE ( 'NONE', #18911, #5453 ) ;
#16718=CARTESIAN_POINT ( 'NONE',  ( 36.31606138205700063, -30.30876147765400574, 73.55501292737010033 ) ) ;
#16719=EDGE_CURVE ( 'NONE', #17700, #7542, #164, .T. ) ;
#16732=EDGE_CURVE ( 'NONE', #13486, #23038, #17771, .T. ) ;
#16738=DIRECTION ( 'NONE',  ( 0.000000000000000000, -1.000000000000000000, 3.115648231731786715E-15 ) ) ;
#16749=CARTESIAN_POINT ( 'NONE',  ( 44.81606138205700063, -38.55876147765400930, 73.30501292737012875 ) ) ;
#16768=DIRECTION ( 'NONE',  ( 0.000000000000000000, 6.938893903907222067E-15, -1.000000000000000000 ) ) ;
#16777=EDGE_CURVE ( 'NONE', #1954, #12862, #6516, .T. ) ;
#16782=EDGE_CURVE ( 'NONE', #21068, #12825, #4830, .T. ) ;
#16786=CARTESIAN_POINT ( 'NONE',  ( 33.56606138205700773, 43.19123852234599781, 75.30501292736987295 ) ) ;
#16789=DIRECTION ( 'NONE',  ( -1.000000000000000000, 0.000000000000000000, 0.000000000000000000 ) ) ;
#16795=ORIENTED_EDGE ( 'NONE', *, *, #8581, .F. ) ;
#16797=CARTESIAN_POINT ( 'NONE',  ( 40.31606138205700773, 37.94123852234599070, 73.55501292736988717 ) ) ;
#16801=ORIENTED_EDGE ( 'NONE', *, *, #15855, .T. ) ;
#16811=ORIENTED_EDGE ( 'NONE', *, *, #21588, .F. ) ;
#16814=EDGE_CURVE ( 'NONE', #4130, #9093, #22388, .T. ) ;
#16816=CARTESIAN_POINT ( 'NONE',  ( 43.81606138205700063, 35.44123852234597649, 68.30501292736990138 ) ) ;
#16825=AXIS2_PLACEMENT_3D ( 'NONE', #22842, #5203, #10999 ) ;
#16828=DIRECTION ( 'NONE',  ( 1.000000000000000000, 0.000000000000000000, 0.000000000000000000 ) ) ;
#16834=ORIENTED_EDGE ( 'NONE', *, *, #18912, .F. ) ;
#16837=LINE ( 'NONE', #16963, #15604 ) ;
#16846=EDGE_CURVE ( 'NONE', #18113, #21608, #17470, .T. ) ;
#16850=VERTEX_POINT ( 'NONE', #17078 ) ;
#16860=ORIENTED_EDGE ( 'NONE', *, *, #19884, .T. ) ;
#16862=CARTESIAN_POINT ( 'NONE',  ( 40.31606138205700773, -30.30876147765399864, 75.30501292736995822 ) ) ;
#16870=AXIS2_PLACEMENT_3D ( 'NONE', #12058, #14234, #2490 ) ;
#16875=CARTESIAN_POINT ( 'NONE',  ( 32.81606138205700773, -38.55876147765401640, 71.30501292737012875 ) ) ;
#16891=CARTESIAN_POINT ( 'NONE',  ( 34.56606138205700773, 42.19123852234599781, 74.30501292736987295 ) ) ;
#16894=CARTESIAN_POINT ( 'NONE',  ( 43.81606138205700063, 28.69846577177642288, 66.12638289304319983 ) ) ;
#16905=ORIENTED_EDGE ( 'NONE', *, *, #18849, .F. ) ;
#16910=AXIS2_PLACEMENT_3D ( 'NONE', #1483, #17596, #5368 ) ;
#16917=DIRECTION ( 'NONE',  ( -1.000000000000000000, 0.000000000000000000, 0.000000000000000000 ) ) ;
#16919=EDGE_CURVE ( 'NONE', #16043, #10464, #13084, .T. ) ;
#16931=LINE ( 'NONE', #15244, #22208 ) ;
#16932=DIRECTION ( 'NONE',  ( 1.000000000000000000, 0.000000000000000000, 0.000000000000000000 ) ) ;
#16934=VERTEX_POINT ( 'NONE', #19755 ) ;
#16938=ORIENTED_EDGE ( 'NONE', *, *, #14937, .F. ) ;
#16942=CARTESIAN_POINT ( 'NONE',  ( 32.81606138205700773, 41.44123852234597649, 67.80501292736988717 ) ) ;
#16945=ORIENTED_EDGE ( 'NONE', *, *, #8620, .T. ) ;
#16960=ORIENTED_EDGE ( 'NONE', *, *, #15205, .T. ) ;
#16963=CARTESIAN_POINT ( 'NONE',  ( 43.81606138205700063, 35.95440708241085304, 61.30501292736990138 ) ) ;
#16965=EDGE_CURVE ( 'NONE', #1363, #21491, #7594, .T. ) ;
#16970=FACE_OUTER_BOUND ( 'NONE', #24003, .T. ) ;
#16976=EDGE_CURVE ( 'NONE', #3140, #5235, #15637, .T. ) ;
#16982=ADVANCED_FACE ( 'NONE', ( #21310 ), #3649, .F. ) ;
#16986=DIRECTION ( 'NONE',  ( -1.000000000000000000, 1.040834085586084551E-30, 3.469446951953615175E-16 ) ) ;
#16989=CYLINDRICAL_SURFACE ( 'NONE', #24618, 1.000000000000000888 ) ;
#16994=VERTEX_POINT ( 'NONE', #21569 ) ;
#16995=ORIENTED_EDGE ( 'NONE', *, *, #3652, .T. ) ;
#16997=VECTOR ( 'NONE', #1699, 1000.000000000000000 ) ;
#16998=PLANE ( 'NONE',  #2540 ) ;
#17002=ORIENTED_EDGE ( 'NONE', *, *, #24940, .T. ) ;
#17003=LINE ( 'NONE', #20480, #5575 ) ;
#17008=CARTESIAN_POINT ( 'NONE',  ( 33.56606138205700773, -34.55876147765400219, 75.30501292737011454 ) ) ;
#17012=CIRCLE ( 'NONE', #1782, 1.750000000000001554 ) ;
#17015=DIRECTION ( 'NONE',  ( -3.717264591378870232E-16, -2.999999999999999839E-15, -1.000000000000000000 ) ) ;
#17035=ORIENTED_EDGE ( 'NONE', *, *, #10520, .T. ) ;
#17036=ORIENTED_EDGE ( 'NONE', *, *, #16782, .T. ) ;
#17048=LINE ( 'NONE', #9676, #22775 ) ;
#17070=ORIENTED_EDGE ( 'NONE', *, *, #6581, .F. ) ;
#17074=CARTESIAN_POINT ( 'NONE',  ( 32.81606138205700773, 41.44123852234599781, 75.30501292736987295 ) ) ;
#17075=ORIENTED_EDGE ( 'NONE', *, *, #24985, .T. ) ;
#17078=CARTESIAN_POINT ( 'NONE',  ( 33.56606138205700773, 42.19123852234599781, 74.30501292736987295 ) ) ;
#17079=CARTESIAN_POINT ( 'NONE',  ( 33.56606138205700773, 43.19123852234595518, 61.30501292736988006 ) ) ;
#17080=VECTOR ( 'NONE', #11756, 1000.000000000000000 ) ;
#17085=VERTEX_POINT ( 'NONE', #10485 ) ;
#17093=ORIENTED_EDGE ( 'NONE', *, *, #978, .T. ) ;
#17111=DIRECTION ( 'NONE',  ( -0.000000000000000000, -1.000000000000000000, 2.999999999999998655E-15 ) ) ;
#17114=ADVANCED_FACE ( 'NONE', ( #18339 ), #4559, .F. ) ;
#17122=FACE_OUTER_BOUND ( 'NONE', #25173, .T. ) ;
#17123=LINE ( 'NONE', #12877, #24282 ) ;
#17124=VERTEX_POINT ( 'NONE', #8425 ) ;
#17130=ORIENTED_EDGE ( 'NONE', *, *, #5951, .F. ) ;
#17139=CARTESIAN_POINT ( 'NONE',  ( 33.56606138205700773, 41.44123852234599781, 74.30501292736987295 ) ) ;
#17144=ADVANCED_FACE ( 'NONE', ( #10105 ), #2228, .F. ) ;
#17145=ORIENTED_EDGE ( 'NONE', *, *, #12501, .F. ) ;
#17151=ADVANCED_FACE ( 'NONE', ( #2720 ), #22320, .T. ) ;
#17154=EDGE_LOOP ( 'NONE', ( #9148, #12711, #10153, #7018 ) ) ;
#17155=CARTESIAN_POINT ( 'NONE',  ( 37.31606138205700063, 43.19123852234595518, 61.30501292736988006 ) ) ;
#17161=VERTEX_POINT ( 'NONE', #4679 ) ;
#17162=DIRECTION ( 'NONE',  ( 9.027796614315171564E-31, 1.000000000000000000, 3.938893903907230117E-15 ) ) ;
#17169=EDGE_CURVE ( 'NONE', #12037, #25254, #412, .T. ) ;
#17177=AXIS2_PLACEMENT_3D ( 'NONE', #384, #10458, #8269 ) ;
#17181=LINE ( 'NONE', #25005, #12237 ) ;
#17185=ORIENTED_EDGE ( 'NONE', *, *, #717, .F. ) ;
#17190=ORIENTED_EDGE ( 'NONE', *, *, #13816, .F. ) ;
#17194=LINE ( 'NONE', #23104, #7771 ) ;
#17197=ADVANCED_FACE ( 'NONE', ( #8167 ), #10227, .F. ) ;
#17204=DIRECTION ( 'NONE',  ( 0.000000000000000000, -1.000000000000000000, 3.965082230804126670E-15 ) ) ;
#17208=CARTESIAN_POINT ( 'NONE',  ( 44.81606138205700063, 41.44123852234599781, 75.30501292736987295 ) ) ;
#17217=AXIS2_PLACEMENT_3D ( 'NONE', #4933, #10989, #24872 ) ;
#17220=ORIENTED_EDGE ( 'NONE', *, *, #22176, .T. ) ;
#17236=DIRECTION ( 'NONE',  ( 0.000000000000000000, 2.775557561562888984E-15, 1.000000000000000000 ) ) ;
#17242=CARTESIAN_POINT ( 'NONE',  ( 35.31606138205687273, 43.19123852234596939, 65.30501292736988717 ) ) ;
#17251=CIRCLE ( 'NONE', #7806, 2.500000000000002220 ) ;
#17252=EDGE_LOOP ( 'NONE', ( #24785, #7776, #22316, #14890, #8280 ) ) ;
#17258=FACE_BOUND ( 'NONE', #17252, .T. ) ;
#17260=CYLINDRICAL_SURFACE ( 'NONE', #12469, 1.750000000000001554 ) ;
#17282=EDGE_CURVE ( 'NONE', #20889, #5342, #7890, .T. ) ;
#17296=CIRCLE ( 'NONE', #10714, 1.750000000000001554 ) ;
#17306=CARTESIAN_POINT ( 'NONE',  ( 32.81606138205700773, 41.44123852234599781, 75.30501292736987295 ) ) ;
#17308=DIRECTION ( 'NONE',  ( -1.000000000000000000, 0.000000000000000000, 0.000000000000000000 ) ) ;
#17315=DIRECTION ( 'NONE',  ( -9.027796614315171564E-31, -1.000000000000000000, -3.938893903907230117E-15 ) ) ;
#17343=EDGE_LOOP ( 'NONE', ( #17379, #10264, #16074, #14421 ) ) ;
#17354=CARTESIAN_POINT ( 'NONE',  ( 39.31606138205700063, 42.19123852234599781, 74.30501292736987295 ) ) ;
#17357=ORIENTED_EDGE ( 'NONE', *, *, #13920, .F. ) ;
#17358=ORIENTED_EDGE ( 'NONE', *, *, #2690, .T. ) ;
#17359=CARTESIAN_POINT ( 'NONE',  ( 36.31606138205700063, 42.19123852234596939, 66.30501292736988717 ) ) ;
#17361=CYLINDRICAL_SURFACE ( 'NONE', #9980, 1.000000000000000888 ) ;
#17372=ORIENTED_EDGE ( 'NONE', *, *, #21996, .F. ) ;
#17375=DIRECTION ( 'NONE',  ( 0.000000000000000000, 1.000000000000000000, -2.999999999999999839E-15 ) ) ;
#17379=ORIENTED_EDGE ( 'NONE', *, *, #4182, .F. ) ;
#17381=CARTESIAN_POINT ( 'NONE',  ( 31.81606138205700418, 38.19123852234598360, 71.05501292736988717 ) ) ;
#17391=AXIS2_PLACEMENT_3D ( 'NONE', #19567, #17776, #15189 ) ;
#17397=CARTESIAN_POINT ( 'NONE',  ( 40.81606138205700773, -31.05876147765399864, 75.30501292737010033 ) ) ;
#17401=EDGE_LOOP ( 'NONE', ( #11609, #21648, #22212, #9748 ) ) ;
#17433=ADVANCED_FACE ( 'NONE', ( #10575 ), #254, .F. ) ;
#17440=VERTEX_POINT ( 'NONE', #22159 ) ;
#17442=ORIENTED_EDGE ( 'NONE', *, *, #5948, .F. ) ;
#17448=ORIENTED_EDGE ( 'NONE', *, *, #21979, .T. ) ;
#17466=AXIS2_PLACEMENT_3D ( 'NONE', #16797, #1333, #20801 ) ;
#17468=ORIENTED_EDGE ( 'NONE', *, *, #13965, .T. ) ;
#17470=CIRCLE ( 'NONE', #4725, 1.000000000000000888 ) ;
#17473=ADVANCED_FACE ( 'NONE', ( #21911 ), #12525, .T. ) ;
#17485=ORIENTED_EDGE ( 'NONE', *, *, #22313, .F. ) ;
#17487=DIRECTION ( 'NONE',  ( 0.000000000000000000, 2.999999999999999839E-15, 1.000000000000000000 ) ) ;
#17495=ORIENTED_EDGE ( 'NONE', *, *, #17637, .T. ) ;
#17504=AXIS2_PLACEMENT_3D ( 'NONE', #5689, #9822, #24202 ) ;
#17507=LINE ( 'NONE', #9903, #21006 ) ;
#17514=ORIENTED_EDGE ( 'NONE', *, *, #25340, .T. ) ;
#17516=LINE ( 'NONE', #25341, #20336 ) ;
#17522=CARTESIAN_POINT ( 'NONE',  ( 40.81606138205700773, -31.05876147765399864, 75.30501292737010033 ) ) ;
#17531=CARTESIAN_POINT ( 'NONE',  ( 40.31606138205700773, -31.05876147765400574, 73.55501292737010033 ) ) ;
#17545=CARTESIAN_POINT ( 'NONE',  ( 36.31606138205700063, -30.30876147765399864, 75.30501292736995822 ) ) ;
#17552=DIRECTION ( 'NONE',  ( 0.000000000000000000, 1.000000000000000000, 0.000000000000000000 ) ) ;
#17553=CARTESIAN_POINT ( 'NONE',  ( 44.81606138205700063, 41.44123852234599070, 73.55501292736987295 ) ) ;
#17565=VERTEX_POINT ( 'NONE', #18806 ) ;
#17573=EDGE_LOOP ( 'NONE', ( #17641, #17870, #2023, #12733 ) ) ;
#17580=ORIENTED_EDGE ( 'NONE', *, *, #20191, .T. ) ;
#17581=EDGE_CURVE ( 'NONE', #14979, #6943, #5861, .T. ) ;
#17588=CARTESIAN_POINT ( 'NONE',  ( 44.81606138205700063, -34.55876147765400930, 73.55501292737011454 ) ) ;
#17590=CARTESIAN_POINT ( 'NONE',  ( 44.81606138205700063, -34.55876147765400930, 73.55501292737011454 ) ) ;
#17593=CARTESIAN_POINT ( 'NONE',  ( 40.81606138205700773, 37.44123852234599781, 74.30501292736988717 ) ) ;
#17596=DIRECTION ( 'NONE',  ( 0.000000000000000000, -2.999999999999999839E-15, -1.000000000000000000 ) ) ;
#17599=LINE ( 'NONE', #7811, #20887 ) ;
#17617=ADVANCED_FACE ( 'NONE', ( #1281 ), #24328, .T. ) ;
#17621=DIRECTION ( 'NONE',  ( 3.491481338843135327E-15, 1.000000000000000000, -2.999999999999999839E-15 ) ) ;
#17623=DIRECTION ( 'NONE',  ( -1.000000000000000000, 0.000000000000000000, 0.000000000000000000 ) ) ;
#17637=EDGE_CURVE ( 'NONE', #18276, #6436, #16480, .T. ) ;
#17640=VECTOR ( 'NONE', #17886, 1000.000000000000000 ) ;
#17641=ORIENTED_EDGE ( 'NONE', *, *, #13741, .T. ) ;
#17647=( NAMED_UNIT ( * ) PLANE_ANGLE_UNIT ( ) SI_UNIT ( $, .RADIAN. ) );
#17649=CARTESIAN_POINT ( 'NONE',  ( 31.81606138205700418, -38.55876147765400930, 73.30501292737012875 ) ) ;
#17650=DIRECTION ( 'NONE',  ( 2.312964634635740294E-15, 2.999999999999999839E-15, 1.000000000000000000 ) ) ;
#17667=DIRECTION ( 'NONE',  ( -1.000000000000000000, 5.204170427930415223E-30, 1.734723475976805122E-15 ) ) ;
#17675=CIRCLE ( 'NONE', #12336, 2.000000000000001776 ) ;
#17683=VECTOR ( 'NONE', #15683, 1000.000000000000000 ) ;
#17699=VERTEX_POINT ( 'NONE', #20067 ) ;
#17700=VERTEX_POINT ( 'NONE', #8602 ) ;
#17701=CARTESIAN_POINT ( 'NONE',  ( 38.31606138205700063, 38.69123852234599070, 72.30501292737018559 ) ) ;
#17712=ORIENTED_EDGE ( 'NONE', *, *, #9813, .T. ) ;
#17724=CARTESIAN_POINT ( 'NONE',  ( 43.81606138205700063, 35.44123852234597649, 67.80501292736990138 ) ) ;
#17725=ORIENTED_EDGE ( 'NONE', *, *, #8620, .F. ) ;
#17734=FACE_OUTER_BOUND ( 'NONE', #7541, .T. ) ;
#17765=EDGE_LOOP ( 'NONE', ( #7281, #1931, #16801, #9307, #7910 ) ) ;
#17767=CYLINDRICAL_SURFACE ( 'NONE', #24752, 1.550000000000002709 ) ;
#17771=LINE ( 'NONE', #16169, #1791 ) ;
#17774=EDGE_CURVE ( 'NONE', #25151, #9366, #14520, .T. ) ;
#17776=DIRECTION ( 'NONE',  ( 1.000000000000000000, -5.510910596163088391E-31, -1.836970198721029688E-16 ) ) ;
#17783=CARTESIAN_POINT ( 'NONE',  ( 32.81606138205700773, -22.55876147765401996, 68.80501292737008612 ) ) ;
#17789=VERTEX_POINT ( 'NONE', #4734 ) ;
#17797=CIRCLE ( 'NONE', #11216, 2.500000000000002220 ) ;
#17801=CARTESIAN_POINT ( 'NONE',  ( 33.56606138205700773, 41.44123852234599070, 73.55501292736987295 ) ) ;
#17809=CIRCLE ( 'NONE', #14920, 1.550000000000002709 ) ;
#17824=VERTEX_POINT ( 'NONE', #18019 ) ;
#17832=CARTESIAN_POINT ( 'NONE',  ( 43.81606138205700063, -34.55876147765403061, 66.30501292737011454 ) ) ;
#17836=VECTOR ( 'NONE', #24617, 1000.000000000000000 ) ;
#17840=EDGE_LOOP ( 'NONE', ( #7433, #5526, #5223, #11354 ) ) ;
#17850=VERTEX_POINT ( 'NONE', #13237 ) ;
#17859=CIRCLE ( 'NONE', #20319, 1.550000000000002709 ) ;
#17860=CARTESIAN_POINT ( 'NONE',  ( 43.81606138205700063, -38.55876147765401640, 71.30501292737012875 ) ) ;
#17866=ORIENTED_EDGE ( 'NONE', *, *, #12634, .F. ) ;
#17867=VERTEX_POINT ( 'NONE', #20571 ) ;
#17870=ORIENTED_EDGE ( 'NONE', *, *, #6530, .T. ) ;
#17871=DIRECTION ( 'NONE',  ( -0.000000000000000000, -1.000000000000000000, 2.848211695852029218E-15 ) ) ;
#17884=DIRECTION ( 'NONE',  ( -1.000000000000000000, 1.115179377413661005E-30, 3.717264591378870232E-16 ) ) ;
#17886=DIRECTION ( 'NONE',  ( 1.000000000000000000, 1.115287202090205222E-30, -1.734723475976805122E-15 ) ) ;
#17891=DIRECTION ( 'NONE',  ( -1.000000000000000000, 1.040834085586084551E-30, 3.469446951953615175E-16 ) ) ;
#17901=ORIENTED_EDGE ( 'NONE', *, *, #16782, .F. ) ;
#17902=CARTESIAN_POINT ( 'NONE',  ( 44.81606138205700063, -38.55876147765400930, 73.30501292737012875 ) ) ;
#17906=DIRECTION ( 'NONE',  ( 0.000000000000000000, 1.000000000000000000, 0.000000000000000000 ) ) ;
#17911=EDGE_CURVE ( 'NONE', #12037, #13486, #24796, .T. ) ;
#17917=EDGE_LOOP ( 'NONE', ( #10637, #2588, #22863, #15776 ) ) ;
#17921=ORIENTED_EDGE ( 'NONE', *, *, #20873, .T. ) ;
#17934=DIRECTION ( 'NONE',  ( 0.000000000000000000, 2.999999999999999839E-15, 1.000000000000000000 ) ) ;
#17935=DIRECTION ( 'NONE',  ( -1.000000000000000000, 0.000000000000000000, 0.000000000000000000 ) ) ;
#17941=EDGE_CURVE ( 'NONE', #12862, #15888, #3168, .T. ) ;
#17954=VERTEX_POINT ( 'NONE', #18896 ) ;
#17958=VERTEX_POINT ( 'NONE', #22627 ) ;
#17960=EDGE_LOOP ( 'NONE', ( #3673, #17002, #2780, #21100 ) ) ;
#17964=CARTESIAN_POINT ( 'NONE',  ( 36.31606138205700063, 38.69123852234599781, 75.30501292737004349 ) ) ;
#17970=DIRECTION ( 'NONE',  ( -1.000000000000000000, 1.040834085586084551E-30, 3.469446951953615175E-16 ) ) ;
#17972=FACE_OUTER_BOUND ( 'NONE', #363, .T. ) ;
#17973=EDGE_LOOP ( 'NONE', ( #6055, #17712, #6654, #21722 ) ) ;
#17977=CARTESIAN_POINT ( 'NONE',  ( 44.81606138205700063, 1.441238522345976714, 67.80501292737001506 ) ) ;
#17982=CARTESIAN_POINT ( 'NONE',  ( 32.81606138205700773, -38.55876147765401640, 70.30501292737012875 ) ) ;
#17991=DIRECTION ( 'NONE',  ( -6.938893903907229955E-15, -1.000000000000000000, 2.999999999999999839E-15 ) ) ;
#17992=DIRECTION ( 'NONE',  ( 0.000000000000000000, -1.000000000000000000, 2.999999999999999839E-15 ) ) ;
#17996=VECTOR ( 'NONE', #18617, 1000.000000000000000 ) ;
#17997=CIRCLE ( 'NONE', #18807, 2.500000000000002220 ) ;
#18003=DIRECTION ( 'NONE',  ( -1.836970198721029688E-16, -2.999999999999999839E-15, -1.000000000000000000 ) ) ;
#18008=DIRECTION ( 'NONE',  ( 0.000000000000000000, 3.469446951953611033E-15, 1.000000000000000000 ) ) ;
#18015=EDGE_LOOP ( 'NONE', ( #19211, #5610, #10903, #6758, #13079, #1290, #12964, #15506, #11431, #5126, #23380, #1589 ) ) ;
#18019=CARTESIAN_POINT ( 'NONE',  ( 43.81606138205700063, 41.44123852234599070, 73.55501292736987295 ) ) ;
#18022=ADVANCED_FACE ( 'NONE', ( #11689 ), #5743, .F. ) ;
#18029=AXIS2_PLACEMENT_3D ( 'NONE', #2273, #10027, #24154 ) ;
#18034=ORIENTED_EDGE ( 'NONE', *, *, #6702, .F. ) ;
#18037=PLANE ( 'NONE',  #15371 ) ;
#18042=DIRECTION ( 'NONE',  ( -1.000000000000000000, -3.083952846180990083E-15, 9.251858538542970050E-30 ) ) ;
#18061=AXIS2_PLACEMENT_3D ( 'NONE', #20279, #18729, #24119 ) ;
#18066=VECTOR ( 'NONE', #9418, 1000.000000000000000 ) ;
#18078=ORIENTED_EDGE ( 'NONE', *, *, #17282, .T. ) ;
#18079=LINE ( 'NONE', #12546, #15628 ) ;
#18084=EDGE_CURVE ( 'NONE', #6775, #16347, #17599, .T. ) ;
#18085=AXIS2_PLACEMENT_3D ( 'NONE', #21137, #5548, #13286 ) ;
#18086=EDGE_LOOP ( 'NONE', ( #842, #12519, #14809, #16268, #3220 ) ) ;
#18091=DIRECTION ( 'NONE',  ( 1.000000000000000000, 0.000000000000000000, 0.000000000000000000 ) ) ;
#18093=LINE ( 'NONE', #8170, #21308 ) ;
#18099=CARTESIAN_POINT ( 'NONE',  ( 33.56606138205700773, 41.44123852234599781, 74.30501292736987295 ) ) ;
#18102=AXIS2_PLACEMENT_3D ( 'NONE', #7067, #14919, #24825 ) ;
#18106=DIRECTION ( 'NONE',  ( 3.053249489819422104E-16, 0.5703958094953464064, 0.8213699656732943444 ) ) ;
#18111=CARTESIAN_POINT ( 'NONE',  ( 32.81606138205700773, 41.44123852234599070, 73.30501292736987295 ) ) ;
#18112=ORIENTED_EDGE ( 'NONE', *, *, #16571, .F. ) ;
#18113=VERTEX_POINT ( 'NONE', #7562 ) ;
#18119=ORIENTED_EDGE ( 'NONE', *, *, #3981, .F. ) ;
#18129=ORIENTED_EDGE ( 'NONE', *, *, #8300, .T. ) ;
#18130=LINE ( 'NONE', #19799, #5479 ) ;
#18134=DIRECTION ( 'NONE',  ( 0.000000000000000000, 1.000000000000000000, -2.999999999999999839E-15 ) ) ;
#18135=AXIS2_PLACEMENT_3D ( 'NONE', #1889, #25199, #5904 ) ;
#18142=LINE ( 'NONE', #14017, #4952 ) ;
#18147=AXIS2_PLACEMENT_3D ( 'NONE', #7949, #570, #949 ) ;
#18148=ORIENTED_EDGE ( 'NONE', *, *, #19631, .F. ) ;
#18158=ADVANCED_FACE ( 'NONE', ( #19270 ), #21459, .T. ) ;
#18163=CARTESIAN_POINT ( 'NONE',  ( 44.81606138205700063, -38.55876147765404482, 61.30501292737012164 ) ) ;
#18169=ORIENTED_EDGE ( 'NONE', *, *, #20456, .T. ) ;
#18175=FACE_OUTER_BOUND ( 'NONE', #17401, .T. ) ;
#18178=ORIENTED_EDGE ( 'NONE', *, *, #11569, .T. ) ;
#18207=VERTEX_POINT ( 'NONE', #20721 ) ;
#18208=DIRECTION ( 'NONE',  ( 0.000000000000000000, -1.000000000000000000, 2.999999999999999839E-15 ) ) ;
#18214=VECTOR ( 'NONE', #22648, 1000.000000000000000 ) ;
#18217=CARTESIAN_POINT ( 'NONE',  ( 36.31606138205700063, -31.05876147765399864, 75.30501292737010033 ) ) ;
#18220=AXIS2_PLACEMENT_3D ( 'NONE', #9879, #9506, #9756 ) ;
#18230=DIRECTION ( 'NONE',  ( -1.000000000000000000, -3.083952846180990083E-15, 9.251858538542970050E-30 ) ) ;
#18236=ORIENTED_EDGE ( 'NONE', *, *, #13741, .F. ) ;
#18238=VECTOR ( 'NONE', #18885, 1000.000000000000000 ) ;
#18239=CARTESIAN_POINT ( 'NONE',  ( 41.81606138205687273, 43.19123852234595518, 61.80501292736988006 ) ) ;
#18246=CIRCLE ( 'NONE', #7127, 1.000000000000000888 ) ;
#18247=CARTESIAN_POINT ( 'NONE',  ( 31.81606138205700418, 38.19123852234599070, 73.05501292736988717 ) ) ;
#18252=EDGE_LOOP ( 'NONE', ( #5432, #7290, #9339, #8379 ) ) ;
#18276=VERTEX_POINT ( 'NONE', #14787 ) ;
#18277=ORIENTED_EDGE ( 'NONE', *, *, #16777, .T. ) ;
#18281=AXIS2_PLACEMENT_3D ( 'NONE', #18685, #6831, #14813 ) ;
#18283=EDGE_CURVE ( 'NONE', #2367, #18444, #16588, .T. ) ;
#18290=DIRECTION ( 'NONE',  ( 1.000000000000000000, 0.000000000000000000, 0.000000000000000000 ) ) ;
#18296=VECTOR ( 'NONE', #9849, 1000.000000000000000 ) ;
#18297=FACE_OUTER_BOUND ( 'NONE', #22686, .T. ) ;
#18306=DIRECTION ( 'NONE',  ( 1.000000000000000000, -1.115179377413661005E-30, -3.717264591378870232E-16 ) ) ;
#18320=DIRECTION ( 'NONE',  ( -1.000000000000000000, 0.000000000000000000, 0.000000000000000000 ) ) ;
#18339=FACE_OUTER_BOUND ( 'NONE', #19160, .T. ) ;
#18357=ORIENTED_EDGE ( 'NONE', *, *, #1826, .F. ) ;
#18358=CARTESIAN_POINT ( 'NONE',  ( 33.56606138205700773, -36.55876147765401640, 71.30501292737011454 ) ) ;
#18359=PLANE ( 'NONE',  #21918 ) ;
#18370=ORIENTED_EDGE ( 'NONE', *, *, #15120, .T. ) ;
#18379=LINE ( 'NONE', #22747, #25477 ) ;
#18394=CARTESIAN_POINT ( 'NONE',  ( 43.81606138205700063, 38.19123852234599070, 72.05501292736988717 ) ) ;
#18412=FACE_OUTER_BOUND ( 'NONE', #19525, .T. ) ;
#18413=LINE ( 'NONE', #15834, #24214 ) ;
#18423=VECTOR ( 'NONE', #16692, 1000.000000000000000 ) ;
#18441=CIRCLE ( 'NONE', #23766, 1.000000000000000888 ) ;
#18444=VERTEX_POINT ( 'NONE', #24930 ) ;
#18456=PLANE ( 'NONE',  #12940 ) ;
#18470=DIRECTION ( 'NONE',  ( -1.000000000000000000, 0.000000000000000000, 0.000000000000000000 ) ) ;
#18476=CARTESIAN_POINT ( 'NONE',  ( 38.31606138205700063, -29.30876147765400930, 72.30501292737010033 ) ) ;
#18483=CARTESIAN_POINT ( 'NONE',  ( 31.81606138205700418, 18.19123852234598715, 71.05501292736995822 ) ) ;
#18497=ORIENTED_EDGE ( 'NONE', *, *, #23804, .F. ) ;
#18504=VECTOR ( 'NONE', #12728, 1000.000000000000000 ) ;
#18505=CARTESIAN_POINT ( 'NONE',  ( 31.81606138205700418, -36.10876147765401356, 70.30501292737011454 ) ) ;
#18510=PLANE ( 'NONE',  #5798 ) ;
#18512=ORIENTED_EDGE ( 'NONE', *, *, #25086, .F. ) ;
#18526=DIRECTION ( 'NONE',  ( -1.000000000000000000, 5.204170427930415223E-30, 1.734723475976805122E-15 ) ) ;
#18536=ORIENTED_EDGE ( 'NONE', *, *, #5951, .T. ) ;
#18538=CARTESIAN_POINT ( 'NONE',  ( 33.56606138205700773, 41.44123852234599070, 73.55501292736987295 ) ) ;
#18539=EDGE_LOOP ( 'NONE', ( #13590, #8529, #16995, #19681, #23938 ) ) ;
#18542=VECTOR ( 'NONE', #16596, 1000.000000000000000 ) ;
#18544=ADVANCED_FACE ( 'NONE', ( #5763 ), #3826, .F. ) ;
#18546=DIRECTION ( 'NONE',  ( 1.000000000000000000, -5.204170427930413997E-31, -1.734723475976804876E-16 ) ) ;
#18555=DIRECTION ( 'NONE',  ( 0.000000000000000000, 1.000000000000000000, -2.999999999999999839E-15 ) ) ;
#18560=AXIS2_PLACEMENT_3D ( 'NONE', #20956, #24668, #20701 ) ;
#18587=EDGE_LOOP ( 'NONE', ( #13828, #9937, #25142, #7622 ) ) ;
#18602=LINE ( 'NONE', #18483, #10877 ) ;
#18605=ORIENTED_EDGE ( 'NONE', *, *, #20753, .T. ) ;
#18607=CARTESIAN_POINT ( 'NONE',  ( 35.31606138205687273, 43.19123852234595518, 61.80501292736988006 ) ) ;
#18617=DIRECTION ( 'NONE',  ( -4.298950768721509852E-32, 1.000000000000000000, -3.115648231731786715E-15 ) ) ;
#18618=ORIENTED_EDGE ( 'NONE', *, *, #24176, .T. ) ;
#18621=CARTESIAN_POINT ( 'NONE',  ( 44.81606138205700063, 41.44123852234599781, 75.30501292736987295 ) ) ;
#18623=CIRCLE ( 'NONE', #19438, 1.750000000000001554 ) ;
#18625=DIRECTION ( 'NONE',  ( 1.734723475976805122E-15, 2.999999999999999839E-15, 1.000000000000000000 ) ) ;
#18627=FACE_OUTER_BOUND ( 'NONE', #23521, .T. ) ;
#18628=ADVANCED_FACE ( 'NONE', ( #21989 ), #11964, .T. ) ;
#18637=ORIENTED_EDGE ( 'NONE', *, *, #19820, .F. ) ;
#18649=CIRCLE ( 'NONE', #10019, 0.7500000000000006661 ) ;
#18663=CARTESIAN_POINT ( 'NONE',  ( 44.81606138205700063, 35.44123852234597649, 67.80501292736990138 ) ) ;
#18671=LINE ( 'NONE', #1010, #13221 ) ;
#18675=EDGE_CURVE ( 'NONE', #3732, #11745, #20054, .T. ) ;
#18681=EDGE_CURVE ( 'NONE', #17958, #10709, #4091, .T. ) ;
#18685=CARTESIAN_POINT ( 'NONE',  ( 32.81606138205700773, 35.95440708241085304, 62.30501292736990138 ) ) ;
#18690=EDGE_CURVE ( 'NONE', #17085, #4130, #20182, .T. ) ;
#18698=LINE ( 'NONE', #22684, #12331 ) ;
#18711=CARTESIAN_POINT ( 'NONE',  ( 32.81606138205700773, -24.55876147765401996, 67.80501292737008612 ) ) ;
#18715=EDGE_CURVE ( 'NONE', #22433, #24927, #21734, .T. ) ;
#18717=DIRECTION ( 'NONE',  ( 0.000000000000000000, 2.775557561562888984E-15, 1.000000000000000000 ) ) ;
#18725=AXIS2_PLACEMENT_3D ( 'NONE', #7753, #15595, #10188 ) ;
#18729=DIRECTION ( 'NONE',  ( -1.000000000000000000, 0.000000000000000000, 0.000000000000000000 ) ) ;
#18734=ORIENTED_EDGE ( 'NONE', *, *, #17169, .T. ) ;
#18744=ORIENTED_EDGE ( 'NONE', *, *, #23926, .T. ) ;
#18749=DIRECTION ( 'NONE',  ( 0.000000000000000000, 1.000000000000000000, 0.000000000000000000 ) ) ;
#18750=ORIENTED_EDGE ( 'NONE', *, *, #20114, .T. ) ;
#18752=ORIENTED_EDGE ( 'NONE', *, *, #796, .T. ) ;
#18778=CARTESIAN_POINT ( 'NONE',  ( 38.31606138205700063, 42.51966564709218233, 71.30501292737018559 ) ) ;
#18779=EDGE_LOOP ( 'NONE', ( #22466, #3574 ) ) ;
#18785=EDGE_CURVE ( 'NONE', #3732, #2891, #2516, .T. ) ;
#18788=ORIENTED_EDGE ( 'NONE', *, *, #22550, .F. ) ;
#18793=UNCERTAINTY_MEASURE_WITH_UNIT (LENGTH_MEASURE( 1.000000000000000082E-05 ), #11924, 'distance_accuracy_value', 'NONE');
#18796=DIRECTION ( 'NONE',  ( 0.000000000000000000, 1.000000000000000000, -2.999999999999999839E-15 ) ) ;
#18800=LINE ( 'NONE', #4890, #10459 ) ;
#18805=DIRECTION ( 'NONE',  ( -1.000000000000000000, 0.000000000000000000, 0.000000000000000000 ) ) ;
#18806=CARTESIAN_POINT ( 'NONE',  ( 32.81606138205700773, -34.55876147765400930, 73.55501292737011454 ) ) ;
#18807=AXIS2_PLACEMENT_3D ( 'NONE', #2236, #17970, #294 ) ;
#18816=CYLINDRICAL_SURFACE ( 'NONE', #10265, 1.550000000000002709 ) ;
#18824=ORIENTED_EDGE ( 'NONE', *, *, #23041, .F. ) ;
#18838=PLANE ( 'NONE',  #22097 ) ;
#18839=DIRECTION ( 'NONE',  ( 0.000000000000000000, -1.000000000000000000, 2.999999999999999839E-15 ) ) ;
#18844=DIRECTION ( 'NONE',  ( 1.000000000000000000, 0.000000000000000000, 0.000000000000000000 ) ) ;
#18845=DIRECTION ( 'NONE',  ( 1.000000000000000000, -3.982629455510873500E-31, -4.336808689942015271E-16 ) ) ;
#18849=EDGE_CURVE ( 'NONE', #11199, #17700, #16429, .T. ) ;
#18852=DIRECTION ( 'NONE',  ( 1.000000000000000000, 2.104045878896135585E-30, -1.734723475976805122E-15 ) ) ;
#18866=ORIENTED_EDGE ( 'NONE', *, *, #3752, .T. ) ;
#18873=EDGE_CURVE ( 'NONE', #4444, #20177, #8724, .T. ) ;
#18875=DIRECTION ( 'NONE',  ( 0.000000000000000000, 1.000000000000000000, -2.999999999999999839E-15 ) ) ;
#18878=ORIENTED_EDGE ( 'NONE', *, *, #15213, .F. ) ;
#18885=DIRECTION ( 'NONE',  ( -7.570943305532639295E-31, -1.000000000000000000, -4.914813388431354887E-16 ) ) ;
#18888=CARTESIAN_POINT ( 'NONE',  ( 41.81606138205687273, 43.19123852234595518, 61.80501292736988006 ) ) ;
#18896=CARTESIAN_POINT ( 'NONE',  ( 43.06606138205700063, 42.19123852234595518, 61.30501292736988006 ) ) ;
#18898=DIRECTION ( 'NONE',  ( 0.000000000000000000, -1.000000000000000000, 2.999999999999999839E-15 ) ) ;
#18900=EDGE_LOOP ( 'NONE', ( #12094, #22986, #24612, #14830 ) ) ;
#18902=DIRECTION ( 'NONE',  ( 1.734723475976805122E-15, 2.999999999999999839E-15, 1.000000000000000000 ) ) ;
#18905=VECTOR ( 'NONE', #20496, 1000.000000000000000 ) ;
#18911=CARTESIAN_POINT ( 'NONE',  ( 40.31606138205700773, -31.05876147765399864, 74.30501292737010033 ) ) ;
#18912=EDGE_CURVE ( 'NONE', #20194, #3140, #15265, .T. ) ;
#18917=AXIS2_PLACEMENT_3D ( 'NONE', #8233, #2416, #2669 ) ;
#18921=AXIS2_PLACEMENT_3D ( 'NONE', #11455, #8312, #18230 ) ;
#18931=DIRECTION ( 'NONE',  ( -1.000000000000000000, 5.204170427930415223E-30, 1.734723475976805122E-15 ) ) ;
#18938=ORIENTED_EDGE ( 'NONE', *, *, #2203, .F. ) ;
#18939=EDGE_CURVE ( 'NONE', #13262, #2806, #18441, .T. ) ;
#18941=CARTESIAN_POINT ( 'NONE',  ( 43.06606138205700063, -36.55876147765401640, 71.30501292737011454 ) ) ;
#18945=EDGE_CURVE ( 'NONE', #17789, #21318, #19013, .T. ) ;
#18948=CARTESIAN_POINT ( 'NONE',  ( 31.81606138205700418, -33.00876147765401925, 70.30501292737011454 ) ) ;
#18951=EDGE_LOOP ( 'NONE', ( #1484, #17190, #11423, #2438 ) ) ;
#18963=CARTESIAN_POINT ( 'NONE',  ( 38.31606138205700063, 39.69123852234598360, 71.30501292737018559 ) ) ;
#18964=VECTOR ( 'NONE', #18546, 1000.000000000000000 ) ;
#18969=VECTOR ( 'NONE', #2115, 1000.000000000000000 ) ;
#18976=DIRECTION ( 'NONE',  ( 0.000000000000000000, -2.999999999999999839E-15, -1.000000000000000000 ) ) ;
#18979=PRODUCT_CONTEXT ( 'NONE', #11795, 'mechanical' ) ;
#18990=ORIENTED_EDGE ( 'NONE', *, *, #24272, .F. ) ;
#18992=DIRECTION ( 'NONE',  ( -1.000000000000000000, 5.204170427930415223E-30, 1.734723475976805122E-15 ) ) ;
#18996=DIRECTION ( 'NONE',  ( 0.000000000000000000, -1.000000000000000000, 2.999999999999999839E-15 ) ) ;
#18998=ORIENTED_EDGE ( 'NONE', *, *, #17774, .T. ) ;
#19002=DIRECTION ( 'NONE',  ( -1.000000000000000000, 0.000000000000000000, 0.000000000000000000 ) ) ;
#19013=LINE ( 'NONE', #15014, #8984 ) ;
#19014=CARTESIAN_POINT ( 'NONE',  ( 44.81606138205700063, 28.12806996228107437, 66.30501292736992980 ) ) ;
#19042=AXIS2_PLACEMENT_3D ( 'NONE', #20820, #24656, #24408 ) ;
#19044=FACE_OUTER_BOUND ( 'NONE', #25332, .T. ) ;
#19046=AXIS2_PLACEMENT_3D ( 'NONE', #11315, #7048, #23133 ) ;
#19069=LINE ( 'NONE', #3211, #10551 ) ;
#19070=VECTOR ( 'NONE', #4564, 1000.000000000000000 ) ;
#19080=LINE ( 'NONE', #10498, #1624 ) ;
#19103=DIRECTION ( 'NONE',  ( -1.000000000000000000, 1.115179377413661005E-30, 3.717264591378870232E-16 ) ) ;
#19105=VECTOR ( 'NONE', #2509, 1000.000000000000000 ) ;
#19107=ORIENTED_EDGE ( 'NONE', *, *, #11536, .T. ) ;
#19111=CARTESIAN_POINT ( 'NONE',  ( 33.56606138205700773, -34.55876147765400930, 73.55501292737011454 ) ) ;
#19122=CARTESIAN_POINT ( 'NONE',  ( 38.31606138205700063, -30.30876147765401285, 71.30501292737010033 ) ) ;
#19135=EDGE_LOOP ( 'NONE', ( #15332, #5462, #13608, #6247, #17070, #15226, #18637, #18866, #21971, #18824, #23057, #2875 ) ) ;
#19146=ORIENTED_EDGE ( 'NONE', *, *, #6443, .T. ) ;
#19147=FACE_OUTER_BOUND ( 'NONE', #22601, .T. ) ;
#19149=ORIENTED_EDGE ( 'NONE', *, *, #23909, .F. ) ;
#19153=ORIENTED_EDGE ( 'NONE', *, *, #24203, .F. ) ;
#19159=EDGE_CURVE ( 'NONE', #11585, #21184, #3060, .T. ) ;
#19160=EDGE_LOOP ( 'NONE', ( #21981, #21898, #8720, #12485 ) ) ;
#19185=LINE ( 'NONE', #5651, #6755 ) ;
#19193=CARTESIAN_POINT ( 'NONE',  ( 31.81606138205700418, 35.95440708241085304, 61.30501292736990138 ) ) ;
#19198=DIRECTION ( 'NONE',  ( 1.000000000000000000, 0.000000000000000000, 0.000000000000000000 ) ) ;
#19205=EDGE_LOOP ( 'NONE', ( #19377, #1429, #12447, #20160 ) ) ;
#19210=CARTESIAN_POINT ( 'NONE',  ( 40.81606138205700773, -31.05876147765399864, 75.30501292737010033 ) ) ;
#19211=ORIENTED_EDGE ( 'NONE', *, *, #2699, .T. ) ;
#19213=CARTESIAN_POINT ( 'NONE',  ( 43.81606138205700063, 35.95440708241085304, 62.30501292736990138 ) ) ;
#19241=VERTEX_POINT ( 'NONE', #7585 ) ;
#19249=ORIENTED_EDGE ( 'NONE', *, *, #4462, .T. ) ;
#19270=FACE_OUTER_BOUND ( 'NONE', #22725, .T. ) ;
#19274=VERTEX_POINT ( 'NONE', #24933 ) ;
#19286=DIRECTION ( 'NONE',  ( 0.000000000000000000, 2.775557561562888984E-15, 1.000000000000000000 ) ) ;
#19287=VECTOR ( 'NONE', #9677, 1000.000000000000000 ) ;
#19294=DIRECTION ( 'NONE',  ( 0.000000000000000000, -1.000000000000000000, 2.999999999999999839E-15 ) ) ;
#19304=DIRECTION ( 'NONE',  ( 0.000000000000000000, 2.848211695852029218E-15, 1.000000000000000000 ) ) ;
#19327=ORIENTED_EDGE ( 'NONE', *, *, #18283, .T. ) ;
#19338=CARTESIAN_POINT ( 'NONE',  ( 32.81606138205700773, -34.55876147765403061, 66.30501292737011454 ) ) ;
#19344=CIRCLE ( 'NONE', #22639, 4.000000000000003553 ) ;
#19364=CARTESIAN_POINT ( 'NONE',  ( 31.81606138205700418, 18.19123852234599426, 73.05501292736995822 ) ) ;
#19377=ORIENTED_EDGE ( 'NONE', *, *, #2925, .F. ) ;
#19379=CARTESIAN_POINT ( 'NONE',  ( 37.31606138205700063, 43.19123852234599781, 74.30501292736987295 ) ) ;
#19382=FACE_OUTER_BOUND ( 'NONE', #4732, .T. ) ;
#19393=CARTESIAN_POINT ( 'NONE',  ( 31.81606138205700418, 38.19123852234598360, 71.05501292736988717 ) ) ;
#19396=EDGE_CURVE ( 'NONE', #12037, #5642, #210, .T. ) ;
#19402=FACE_OUTER_BOUND ( 'NONE', #18900, .T. ) ;
#19404=CARTESIAN_POINT ( 'NONE',  ( 38.31606138205700063, 42.51966564709218233, 70.30501292737018559 ) ) ;
#19417=DIRECTION ( 'NONE',  ( 0.000000000000000000, -2.999999999999999839E-15, -1.000000000000000000 ) ) ;
#19429=ORIENTED_EDGE ( 'NONE', *, *, #16732, .F. ) ;
#19436=LINE ( 'NONE', #17649, #20322 ) ;
#19437=CARTESIAN_POINT ( 'NONE',  ( 34.56606138205700773, 43.19123852234599781, 75.30501292736987295 ) ) ;
#19438=AXIS2_PLACEMENT_3D ( 'NONE', #20844, #18526, #9001 ) ;
#19443=ORIENTED_EDGE ( 'NONE', *, *, #479, .F. ) ;
#19446=CARTESIAN_POINT ( 'NONE',  ( 44.81606138205700063, -38.55876147765401640, 70.30501292737012875 ) ) ;
#19447=ORIENTED_EDGE ( 'NONE', *, *, #12413, .F. ) ;
#19461=ORIENTED_EDGE ( 'NONE', *, *, #21210, .F. ) ;
#19463=FACE_OUTER_BOUND ( 'NONE', #25409, .T. ) ;
#19464=LINE ( 'NONE', #21273, #21545 ) ;
#19479=VECTOR ( 'NONE', #103, 1000.000000000000000 ) ;
#19490=EDGE_CURVE ( 'NONE', #23735, #6436, #11463, .T. ) ;
#19491=AXIS2_PLACEMENT_3D ( 'NONE', #14565, #2954, #18320 ) ;
#19497=ORIENTED_EDGE ( 'NONE', *, *, #4182, .T. ) ;
#19498=VERTEX_POINT ( 'NONE', #16432 ) ;
#19501=ORIENTED_EDGE ( 'NONE', *, *, #17581, .F. ) ;
#19512=DIRECTION ( 'NONE',  ( 0.000000000000000000, -1.000000000000000000, 2.999999999999999839E-15 ) ) ;
#19525=EDGE_LOOP ( 'NONE', ( #9303, #21620, #8451, #16193 ) ) ;
#19526=ORIENTED_EDGE ( 'NONE', *, *, #17911, .T. ) ;
#19533=CYLINDRICAL_SURFACE ( 'NONE', #8693, 1.000000000000000888 ) ;
#19548=ADVANCED_FACE ( 'NONE', ( #18627 ), #12973, .T. ) ;
#19549=CARTESIAN_POINT ( 'NONE',  ( 31.81606138205700418, -36.55876147765401640, 71.30501292737011454 ) ) ;
#19558=ORIENTED_EDGE ( 'NONE', *, *, #12228, .F. ) ;
#19562=DIRECTION ( 'NONE',  ( -1.000000000000000000, 5.204170427930413997E-31, 1.734723475976804876E-16 ) ) ;
#19565=VERTEX_POINT ( 'NONE', #6907 ) ;
#19567=CARTESIAN_POINT ( 'NONE',  ( 40.81606138205700773, -31.05876147765399864, 75.30501292737010033 ) ) ;
#19577=DIRECTION ( 'NONE',  ( 1.000000000000000000, -5.204170427930415223E-30, -1.734723475976805122E-15 ) ) ;
#19578=FACE_OUTER_BOUND ( 'NONE', #19205, .T. ) ;
#19580=ORIENTED_EDGE ( 'NONE', *, *, #18675, .F. ) ;
#19604=CARTESIAN_POINT ( 'NONE',  ( 32.81606138205700773, -36.55876147765401640, 71.30501292737011454 ) ) ;
#19615=ORIENTED_EDGE ( 'NONE', *, *, #20927, .F. ) ;
#19631=EDGE_CURVE ( 'NONE', #5023, #13361, #20318, .T. ) ;
#19646=ORIENTED_EDGE ( 'NONE', *, *, #12267, .T. ) ;
#19647=EDGE_LOOP ( 'NONE', ( #9106, #1198, #13751, #7565 ) ) ;
#19652=AXIS2_PLACEMENT_3D ( 'NONE', #22041, #6457, #20237 ) ;
#19666=ORIENTED_EDGE ( 'NONE', *, *, #5647, .T. ) ;
#19667=VERTEX_POINT ( 'NONE', #17590 ) ;
#19668=DIRECTION ( 'NONE',  ( -3.373073425510455500E-16, -2.999999999999999839E-15, -1.000000000000000000 ) ) ;
#19671=LINE ( 'NONE', #7966, #15726 ) ;
#19672=VECTOR ( 'NONE', #25282, 1000.000000000000000 ) ;
#19681=ORIENTED_EDGE ( 'NONE', *, *, #6906, .F. ) ;
#19684=CARTESIAN_POINT ( 'NONE',  ( 39.31606138205700063, 42.19123852234596939, 66.30501292736988717 ) ) ;
#19694=DIRECTION ( 'NONE',  ( 9.027796614315171564E-31, 1.000000000000000000, 1.163336342344340343E-15 ) ) ;
#19695=FACE_OUTER_BOUND ( 'NONE', #4470, .T. ) ;
#19698=CARTESIAN_POINT ( 'NONE',  ( 42.06606138205700063, 43.19123852234599781, 74.30501292736987295 ) ) ;
#19712=DIRECTION ( 'NONE',  ( -1.000000000000000000, 5.204170427930413997E-31, 1.734723475976804876E-16 ) ) ;
#19716=DIRECTION ( 'NONE',  ( 8.673617379884039170E-17, 2.999999999999999839E-15, 1.000000000000000000 ) ) ;
#19720=DIRECTION ( 'NONE',  ( -4.812258323195720155E-32, 1.000000000000000000, -3.129456975819164530E-15 ) ) ;
#19728=AXIS2_PLACEMENT_3D ( 'NONE', #16281, #24127, #6504 ) ;
#19734=AXIS2_PLACEMENT_3D ( 'NONE', #5489, #15142, #22997 ) ;
#19738=CARTESIAN_POINT ( 'NONE',  ( 39.31606138205700063, 43.19123852234596939, 66.30501292736988717 ) ) ;
#19748=ORIENTED_EDGE ( 'NONE', *, *, #17774, .F. ) ;
#19755=CARTESIAN_POINT ( 'NONE',  ( 32.81606138205700773, 18.19123852234598715, 71.05501292736995822 ) ) ;
#19770=CIRCLE ( 'NONE', #18135, 1.750000000000001554 ) ;
#19798=ORIENTED_EDGE ( 'NONE', *, *, #5702, .F. ) ;
#19799=CARTESIAN_POINT ( 'NONE',  ( 40.81606138205700773, 37.44123852234599781, 75.30501292736990138 ) ) ;
#19802=DIRECTION ( 'NONE',  ( 0.000000000000000000, -1.000000000000000000, 2.999999999999999839E-15 ) ) ;
#19817=AXIS2_PLACEMENT_3D ( 'NONE', #22062, #23859, #4426 ) ;
#19818=DIRECTION ( 'NONE',  ( -3.491481338843135327E-15, -1.000000000000000000, 2.999999999999999839E-15 ) ) ;
#19820=EDGE_CURVE ( 'NONE', #5864, #12889, #6117, .T. ) ;
#19825=CARTESIAN_POINT ( 'NONE',  ( 43.81606138205700063, 18.19123852234599070, 72.05501292736995822 ) ) ;
#19837=EDGE_CURVE ( 'NONE', #3712, #3791, #23635, .T. ) ;
#19848=VERTEX_POINT ( 'NONE', #21701 ) ;
#19849=CARTESIAN_POINT ( 'NONE',  ( 40.81606138205700773, 37.44123852234599781, 75.30501292736990138 ) ) ;
#19850=CARTESIAN_POINT ( 'NONE',  ( 43.81606138205700063, -34.55876147765401640, 70.30501292737011454 ) ) ;
#19851=AXIS2_PLACEMENT_3D ( 'NONE', #317, #24264, #14369 ) ;
#19856=LINE ( 'NONE', #4400, #3961 ) ;
#19862=AXIS2_PLACEMENT_3D ( 'NONE', #11160, #16430, #18625 ) ;
#19864=DIRECTION ( 'NONE',  ( 0.000000000000000000, 3.469446951953611033E-15, 1.000000000000000000 ) ) ;
#19884=EDGE_CURVE ( 'NONE', #3466, #16707, #10116, .T. ) ;
#19891=AXIS2_PLACEMENT_3D ( 'NONE', #24988, #5684, #9440 ) ;
#19899=FILL_AREA_STYLE ('',( #21824 ) ) ;
#19912=LINE ( 'NONE', #23885, #14384 ) ;
#19927=CIRCLE ( 'NONE', #3474, 1.000000000000000888 ) ;
#19933=CARTESIAN_POINT ( 'NONE',  ( 31.81606138205700418, 28.69846577177642288, 66.12638289304319983 ) ) ;
#19939=LINE ( 'NONE', #16064, #11161 ) ;
#19942=AXIS2_PLACEMENT_3D ( 'NONE', #10605, #8678, #16510 ) ;
#19955=ORIENTED_EDGE ( 'NONE', *, *, #14374, .F. ) ;
#19956=AXIS2_PLACEMENT_3D ( 'NONE', #9156, #20741, #3077 ) ;
#19959=EDGE_CURVE ( 'NONE', #9905, #10647, #15897, .T. ) ;
#19964=DIRECTION ( 'NONE',  ( 0.000000000000000000, 2.999999999999999839E-15, 1.000000000000000000 ) ) ;
#19967=ORIENTED_EDGE ( 'NONE', *, *, #1376, .T. ) ;
#19969=LINE ( 'NONE', #8630, #11983 ) ;
#19970=ORIENTED_EDGE ( 'NONE', *, *, #16732, .T. ) ;
#19971=ORIENTED_EDGE ( 'NONE', *, *, #3670, .F. ) ;
#19977=EDGE_CURVE ( 'NONE', #1424, #4665, #6617, .T. ) ;
#19988=DIRECTION ( 'NONE',  ( 1.000000000000000000, -5.204170427930415223E-30, -1.734723475976805122E-15 ) ) ;
#19990=DIRECTION ( 'NONE',  ( 1.000000000000000000, -1.301042606982604506E-30, -4.336808689942015271E-16 ) ) ;
#20013=CARTESIAN_POINT ( 'NONE',  ( 40.81606138205700773, -24.05876147765399864, 75.30501292737008612 ) ) ;
#20014=EDGE_CURVE ( 'NONE', #17850, #3732, #23391, .T. ) ;
#20029=ORIENTED_EDGE ( 'NONE', *, *, #5176, .F. ) ;
#20039=ORIENTED_EDGE ( 'NONE', *, *, #9826, .T. ) ;
#20040=DIRECTION ( 'NONE',  ( 0.000000000000000000, 1.000000000000000000, 0.000000000000000000 ) ) ;
#20043=EDGE_CURVE ( 'NONE', #13011, #3712, #5314, .T. ) ;
#20045=VECTOR ( 'NONE', #9984, 1000.000000000000000 ) ;
#20052=DIRECTION ( 'NONE',  ( 0.000000000000000000, 1.000000000000000000, 0.000000000000000000 ) ) ;
#20054=LINE ( 'NONE', #328, #10616 ) ;
#20055=FACE_BOUND ( 'NONE', #25167, .T. ) ;
#20061=DIRECTION ( 'NONE',  ( 0.000000000000000000, -3.965082230804126670E-15, -1.000000000000000000 ) ) ;
#20065=ORIENTED_EDGE ( 'NONE', *, *, #18912, .T. ) ;
#20067=CARTESIAN_POINT ( 'NONE',  ( 44.81606138205700063, -34.55876147765400930, 73.30501292737011454 ) ) ;
#20085=VERTEX_POINT ( 'NONE', #4571 ) ;
#20094=DIRECTION ( 'NONE',  ( 3.717264591378870232E-16, 3.115648231731786715E-15, 1.000000000000000000 ) ) ;
#20095=AXIS2_PLACEMENT_3D ( 'NONE', #15318, #7724, #11596 ) ;
#20114=EDGE_CURVE ( 'NONE', #9377, #16043, #932, .T. ) ;
#20133=ORIENTED_EDGE ( 'NONE', *, *, #16265, .T. ) ;
#20139=ADVANCED_FACE ( 'NONE', ( #8823 ), #14851, .F. ) ;
#20145=VECTOR ( 'NONE', #6173, 1000.000000000000000 ) ;
#20150=CARTESIAN_POINT ( 'NONE',  ( 38.31606138205712853, 43.19123852234599781, 75.30501292736987295 ) ) ;
#20152=DIRECTION ( 'NONE',  ( 6.195440985631459015E-17, 1.000000000000000000, -2.999999999999999839E-15 ) ) ;
#20155=AXIS2_PLACEMENT_3D ( 'NONE', #11041, #18898, #4581 ) ;
#20160=ORIENTED_EDGE ( 'NONE', *, *, #22134, .F. ) ;
#20167=ORIENTED_EDGE ( 'NONE', *, *, #13046, .T. ) ;
#20173=CARTESIAN_POINT ( 'NONE',  ( 40.31606138205700773, -30.30876147765400574, 73.55501292737010033 ) ) ;
#20176=VERTEX_POINT ( 'NONE', #22586 ) ;
#20177=VERTEX_POINT ( 'NONE', #6494 ) ;
#20182=LINE ( 'NONE', #4216, #13901 ) ;
#20184=CIRCLE ( 'NONE', #9090, 0.7500000000000006661 ) ;
#20191=EDGE_CURVE ( 'NONE', #20177, #13483, #9457, .T. ) ;
#20194=VERTEX_POINT ( 'NONE', #15360 ) ;
#20197=CIRCLE ( 'NONE', #15239, 1.000000000000000888 ) ;
#20206=DIRECTION ( 'NONE',  ( 0.000000000000000000, 1.000000000000000000, 0.000000000000000000 ) ) ;
#20207=DIRECTION ( 'NONE',  ( -1.000000000000000000, 0.000000000000000000, 0.000000000000000000 ) ) ;
#20208=CARTESIAN_POINT ( 'NONE',  ( 40.31606138205700773, 43.19123852234599781, 75.30501292736987295 ) ) ;
#20210=DIRECTION ( 'NONE',  ( -0.000000000000000000, -1.000000000000000000, 2.848211695852029218E-15 ) ) ;
#20215=VERTEX_POINT ( 'NONE', #15108 ) ;
#20227=CARTESIAN_POINT ( 'NONE',  ( 32.81606138205700773, 41.44123852234596939, 66.30501292736988717 ) ) ;
#20237=DIRECTION ( 'NONE',  ( 0.000000000000000000, 1.000000000000000000, 0.000000000000000000 ) ) ;
#20245=VECTOR ( 'NONE', #16206, 1000.000000000000000 ) ;
#20271=CARTESIAN_POINT ( 'NONE',  ( 44.81606138205700063, -24.55876147765401285, 70.30501292737008612 ) ) ;
#20272=VECTOR ( 'NONE', #24017, 1000.000000000000000 ) ;
#20279=CARTESIAN_POINT ( 'NONE',  ( 43.81606138205700063, -36.55876147765401640, 71.30501292737011454 ) ) ;
#20285=ADVANCED_FACE ( 'NONE', ( #21289 ), #1689, .T. ) ;
#20288=VECTOR ( 'NONE', #15624, 1000.000000000000000 ) ;
#20308=LINE ( 'NONE', #23777, #1926 ) ;
#20311=VERTEX_POINT ( 'NONE', #1452 ) ;
#20317=DIRECTION ( 'NONE',  ( 0.000000000000000000, -2.999999999999999839E-15, -1.000000000000000000 ) ) ;
#20318=LINE ( 'NONE', #18505, #7761 ) ;
#20319=AXIS2_PLACEMENT_3D ( 'NONE', #19850, #12140, #10189 ) ;
#20322=VECTOR ( 'NONE', #7253, 1000.000000000000000 ) ;
#20324=VERTEX_POINT ( 'NONE', #25002 ) ;
#20336=VECTOR ( 'NONE', #13268, 1000.000000000000000 ) ;
#20344=DIRECTION ( 'NONE',  ( -1.000000000000000000, 0.000000000000000000, 0.000000000000000000 ) ) ;
#20355=DIRECTION ( 'NONE',  ( 1.734723475976804876E-16, -1.163336342344335610E-15, 1.000000000000000000 ) ) ;
#20373=EDGE_CURVE ( 'NONE', #22901, #20176, #2412, .T. ) ;
#20375=VECTOR ( 'NONE', #16738, 1000.000000000000000 ) ;
#20379=ORIENTED_EDGE ( 'NONE', *, *, #881, .T. ) ;
#20387=DIRECTION ( 'NONE',  ( 0.000000000000000000, -2.999999999999999839E-15, -1.000000000000000000 ) ) ;
#20395=DIRECTION ( 'NONE',  ( 0.000000000000000000, 1.000000000000000000, 0.000000000000000000 ) ) ;
#20409=FACE_OUTER_BOUND ( 'NONE', #11239, .T. ) ;
#20431=ORIENTED_EDGE ( 'NONE', *, *, #21284, .F. ) ;
#20445=AXIS2_PLACEMENT_3D ( 'NONE', #22324, #18839, #9071 ) ;
#20456=EDGE_CURVE ( 'NONE', #8796, #6972, #17675, .T. ) ;
#20466=ORIENTED_EDGE ( 'NONE', *, *, #16478, .F. ) ;
#20472=EDGE_CURVE ( 'NONE', #17699, #3791, #2329, .T. ) ;
#20480=CARTESIAN_POINT ( 'NONE',  ( 31.81606138205700418, 39.19123852234599070, 72.05501292736988717 ) ) ;
#20481=DIRECTION ( 'NONE',  ( 0.000000000000000000, -1.000000000000000000, 2.999999999999999839E-15 ) ) ;
#20496=DIRECTION ( 'NONE',  ( 0.000000000000000000, -1.000000000000000000, 2.999999999999999839E-15 ) ) ;
#20506=EDGE_LOOP ( 'NONE', ( #1831, #9464, #20065, #3576 ) ) ;
#20510=LINE ( 'NONE', #10857, #10613 ) ;
#20525=CARTESIAN_POINT ( 'NONE',  ( 31.81606138205700418, 35.95440708241085304, 62.30501292736990138 ) ) ;
#20532=ORIENTED_EDGE ( 'NONE', *, *, #21227, .F. ) ;
#20537=DIRECTION ( 'NONE',  ( 0.000000000000000000, 2.999999999999999839E-15, 1.000000000000000000 ) ) ;
#20544=DIRECTION ( 'NONE',  ( 0.000000000000000000, 0.000000000000000000, 1.000000000000000000 ) ) ;
#20552=ORIENTED_EDGE ( 'NONE', *, *, #2778, .F. ) ;
#20555=AXIS2_PLACEMENT_3D ( 'NONE', #116, #17891, #13532 ) ;
#20558=DIRECTION ( 'NONE',  ( -2.120312145707929538E-16, 0.8213699656732942334, -0.5703958094953462954 ) ) ;
#20559=LINE ( 'NONE', #8725, #18238 ) ;
#20565=LINE ( 'NONE', #10659, #2790 ) ;
#20569=ORIENTED_EDGE ( 'NONE', *, *, #2098, .T. ) ;
#20571=CARTESIAN_POINT ( 'NONE',  ( 41.31606138205687273, 42.19123852234596939, 65.30501292736988717 ) ) ;
#20575=ORIENTED_EDGE ( 'NONE', *, *, #20753, .F. ) ;
#20596=DIRECTION ( 'NONE',  ( 0.000000000000000000, 1.000000000000000000, -2.999999999999999839E-15 ) ) ;
#20608=CARTESIAN_POINT ( 'NONE',  ( 40.31606138205700773, -29.30876147765400219, 74.30501292737010033 ) ) ;
#20611=DIRECTION ( 'NONE',  ( -1.000000000000000000, 0.000000000000000000, 0.000000000000000000 ) ) ;
#20629=EDGE_CURVE ( 'NONE', #5882, #13733, #13550, .T. ) ;
#20634=ORIENTED_EDGE ( 'NONE', *, *, #2925, .T. ) ;
#20639=DIRECTION ( 'NONE',  ( 0.000000000000000000, 0.000000000000000000, 1.000000000000000000 ) ) ;
#20646=CARTESIAN_POINT ( 'NONE',  ( 43.06606138205700063, 43.19123852234595518, 61.30501292736988006 ) ) ;
#20650=CARTESIAN_POINT ( 'NONE',  ( 36.31606138205700063, 39.69123852234597649, 69.30501292736988717 ) ) ;
#20674=CARTESIAN_POINT ( 'NONE',  ( 31.81606138205700418, 18.19123852234599070, 72.05501292736995822 ) ) ;
#20682=EDGE_LOOP ( 'NONE', ( #10648, #15840, #24635, #5004 ) ) ;
#20687=DIRECTION ( 'NONE',  ( 1.000000000000000000, 0.000000000000000000, 0.000000000000000000 ) ) ;
#20694=VECTOR ( 'NONE', #7034, 1000.000000000000000 ) ;
#20700=EDGE_CURVE ( 'NONE', #13391, #2408, #12655, .T. ) ;
#20701=DIRECTION ( 'NONE',  ( 0.000000000000000000, 1.000000000000000000, 0.000000000000000000 ) ) ;
#20705=DIRECTION ( 'NONE',  ( -1.000000000000000000, 0.000000000000000000, 0.000000000000000000 ) ) ;
#20721=CARTESIAN_POINT ( 'NONE',  ( 44.81606138205700063, -34.55876147765403061, 66.30501292737011454 ) ) ;
#20727=ORIENTED_EDGE ( 'NONE', *, *, #16044, .T. ) ;
#20741=DIRECTION ( 'NONE',  ( -6.938893903907229955E-15, 1.000000000000000000, -2.999999999999999050E-15 ) ) ;
#20749=EDGE_CURVE ( 'NONE', #15791, #9810, #9424, .T. ) ;
#20753=EDGE_CURVE ( 'NONE', #8442, #16850, #4106, .T. ) ;
#20756=AXIS2_PLACEMENT_3D ( 'NONE', #541, #663, #16382 ) ;
#20760=DIRECTION ( 'NONE',  ( -1.000000000000000000, 0.000000000000000000, 0.000000000000000000 ) ) ;
#20762=ORIENTED_EDGE ( 'NONE', *, *, #15213, .T. ) ;
#20763=EDGE_CURVE ( 'NONE', #13486, #11800, #3480, .T. ) ;
#20765=DIRECTION ( 'NONE',  ( 3.491481338843135327E-15, -1.000000000000000000, 2.999999999999999839E-15 ) ) ;
#20766=COLOUR_RGB ( '', 0.31764706, 0.68627451, 0.89019608) ;
#20785=ORIENTED_EDGE ( 'NONE', *, *, #11536, .F. ) ;
#20789=CIRCLE ( 'NONE', #2672, 1.550000000000002709 ) ;
#20792=AXIS2_PLACEMENT_3D ( 'NONE', #23833, #22287, #10322 ) ;
#20801=DIRECTION ( 'NONE',  ( 1.734723475976805122E-15, 2.999999999999999839E-15, 1.000000000000000000 ) ) ;
#20807=DIRECTION ( 'NONE',  ( 1.000000000000000000, 0.000000000000000000, 0.000000000000000000 ) ) ;
#20808=DIRECTION ( 'NONE',  ( -1.000000000000000000, 1.115179377413661005E-30, 3.717264591378870232E-16 ) ) ;
#20812=ADVANCED_FACE ( 'NONE', ( #12908 ), #7352, .F. ) ;
#20820=CARTESIAN_POINT ( 'NONE',  ( 40.31606138205700773, 39.69123852234597649, 69.30501292736988717 ) ) ;
#20824=CARTESIAN_POINT ( 'NONE',  ( 40.31606138205700773, 37.94123852234599781, 75.30501292736988717 ) ) ;
#20835=EDGE_CURVE ( 'NONE', #6972, #4199, #1656, .T. ) ;
#20836=ORIENTED_EDGE ( 'NONE', *, *, #3487, .T. ) ;
#20843=ORIENTED_EDGE ( 'NONE', *, *, #10358, .F. ) ;
#20844=CARTESIAN_POINT ( 'NONE',  ( 36.31606138205700063, -31.05876147765400574, 73.55501292737010033 ) ) ;
#20845=ADVANCED_FACE ( 'NONE', ( #13028 ), #18816, .F. ) ;
#20861=ORIENTED_EDGE ( 'NONE', *, *, #24497, .T. ) ;
#20873=EDGE_CURVE ( 'NONE', #21126, #15455, #24625, .T. ) ;
#20880=CARTESIAN_POINT ( 'NONE',  ( 41.81606138205687273, 42.19123852234595518, 61.80501292736988006 ) ) ;
#20886=VECTOR ( 'NONE', #23327, 1000.000000000000000 ) ;
#20887=VECTOR ( 'NONE', #1988, 1000.000000000000000 ) ;
#20889=VERTEX_POINT ( 'NONE', #15074 ) ;
#20893=EDGE_CURVE ( 'NONE', #21703, #22091, #9060, .T. ) ;
#20905=ADVANCED_FACE ( 'NONE', ( #7870 ), #3729, .F. ) ;
#20909=VECTOR ( 'NONE', #19802, 1000.000000000000000 ) ;
#20922=ORIENTED_EDGE ( 'NONE', *, *, #11446, .T. ) ;
#20927=EDGE_CURVE ( 'NONE', #21068, #3466, #24244, .T. ) ;
#20928=AXIS2_PLACEMENT_3D ( 'NONE', #966, #16695, #4728 ) ;
#20956=CARTESIAN_POINT ( 'NONE',  ( 44.81606138205700063, -34.55876147765401640, 70.30501292737011454 ) ) ;
#20961=DIRECTION ( 'NONE',  ( 0.000000000000000000, -1.000000000000000000, 2.999999999999999839E-15 ) ) ;
#20965=CARTESIAN_POINT ( 'NONE',  ( 40.31606138205700773, 39.69123852234599781, 74.30501292736988717 ) ) ;
#20966=CARTESIAN_POINT ( 'NONE',  ( 41.31606138205687273, 42.19123852234595518, 61.80501292736988006 ) ) ;
#20969=CARTESIAN_POINT ( 'NONE',  ( 31.81606138205700418, 28.12806996228107081, 65.30501292736992980 ) ) ;
#20972=CIRCLE ( 'NONE', #1225, 1.000000000000000888 ) ;
#20977=LINE ( 'NONE', #15167, #18214 ) ;
#20982=CARTESIAN_POINT ( 'NONE',  ( 36.31606138205703616, 33.19123852234596939, 66.30501292736991559 ) ) ;
#21003=AXIS2_PLACEMENT_3D ( 'NONE', #12791, #21022, #5303 ) ;
#21004=CARTESIAN_POINT ( 'NONE',  ( 40.31606138205700773, 37.94123852234599781, 74.30501292736988717 ) ) ;
#21006=VECTOR ( 'NONE', #19294, 1000.000000000000000 ) ;
#21021=ORIENTED_EDGE ( 'NONE', *, *, #22216, .F. ) ;
#21022=DIRECTION ( 'NONE',  ( -1.000000000000000000, 1.040834085586084551E-30, 3.469446951953615175E-16 ) ) ;
#21037=CYLINDRICAL_SURFACE ( 'NONE', #2561, 1.000000000000000888 ) ;
#21044=VECTOR ( 'NONE', #21601, 1000.000000000000000 ) ;
#21047=ADVANCED_FACE ( 'NONE', ( #2427 ), #12625, .T. ) ;
#21059=CARTESIAN_POINT ( 'NONE',  ( 43.81606138205700063, 28.12806996228107437, 66.30501292736992980 ) ) ;
#21068=VERTEX_POINT ( 'NONE', #8376 ) ;
#21070=EDGE_CURVE ( 'NONE', #8317, #16702, #11109, .T. ) ;
#21084=VERTEX_POINT ( 'NONE', #24939 ) ;
#21096=LINE ( 'NONE', #9381, #21887 ) ;
#21097=ADVANCED_FACE ( 'NONE', ( #17122 ), #13003, .F. ) ;
#21100=ORIENTED_EDGE ( 'NONE', *, *, #22176, .F. ) ;
#21108=DIRECTION ( 'NONE',  ( 0.000000000000000000, 1.000000000000000000, 0.000000000000000000 ) ) ;
#21118=DIRECTION ( 'NONE',  ( 1.836970198721029688E-16, 2.999999999999999839E-15, 1.000000000000000000 ) ) ;
#21123=DIRECTION ( 'NONE',  ( 1.000000000000000000, 0.000000000000000000, 0.000000000000000000 ) ) ;
#21126=VERTEX_POINT ( 'NONE', #1394 ) ;
#21137=CARTESIAN_POINT ( 'NONE',  ( 43.06606138205700063, 41.44123852234599070, 73.55501292736987295 ) ) ;
#21148=ADVANCED_FACE ( 'NONE', ( #3324 ), #11065, .F. ) ;
#21151=PLANE ( 'NONE',  #23329 ) ;
#21170=PRODUCT_DEFINITION_FORMATION_WITH_SPECIFIED_SOURCE ( 'ANY', '', #9311, .NOT_KNOWN. ) ;
#21172=AXIS2_PLACEMENT_3D ( 'NONE', #13829, #9472, #25399 ) ;
#21176=ORIENTED_EDGE ( 'NONE', *, *, #1180, .T. ) ;
#21183=ORIENTED_EDGE ( 'NONE', *, *, #4197, .T. ) ;
#21184=VERTEX_POINT ( 'NONE', #13388 ) ;
#21185=DIRECTION ( 'NONE',  ( 0.000000000000000000, 1.000000000000000000, 0.000000000000000000 ) ) ;
#21186=CARTESIAN_POINT ( 'NONE',  ( 41.81606138205687273, 42.19123852234595518, 61.30501292736988006 ) ) ;
#21191=LINE ( 'NONE', #7413, #712 ) ;
#21195=CARTESIAN_POINT ( 'NONE',  ( 40.81606138205700773, -31.05876147765399864, 75.30501292737010033 ) ) ;
#21210=EDGE_CURVE ( 'NONE', #6943, #25358, #23028, .T. ) ;
#21227=EDGE_CURVE ( 'NONE', #18113, #18276, #5006, .T. ) ;
#21238=CARTESIAN_POINT ( 'NONE',  ( 38.31606138205687984, 42.19123852234596939, 65.30501292736988717 ) ) ;
#21241=EDGE_CURVE ( 'NONE', #18444, #4444, #8650, .T. ) ;
#21245=DIRECTION ( 'NONE',  ( 6.195440985631459015E-17, 1.000000000000000000, -2.999999999999999839E-15 ) ) ;
#21249=CARTESIAN_POINT ( 'NONE',  ( 40.31606138205700773, 39.69123852234599781, 74.30501292736988717 ) ) ;
#21251=LINE ( 'NONE', #9795, #22576 ) ;
#21259=EDGE_LOOP ( 'NONE', ( #10693, #18119, #18938, #1576 ) ) ;
#21265=CARTESIAN_POINT ( 'NONE',  ( 43.81606138205700063, -36.10876147765401356, 70.30501292737011454 ) ) ;
#21273=CARTESIAN_POINT ( 'NONE',  ( 43.06606138205700063, 42.19123852234599070, 73.55501292736987295 ) ) ;
#21284=EDGE_CURVE ( 'NONE', #11368, #21068, #24122, .T. ) ;
#21289=FACE_OUTER_BOUND ( 'NONE', #15850, .T. ) ;
#21297=CARTESIAN_POINT ( 'NONE',  ( 35.81606138205700063, 41.44123852234599781, 75.30501292736988717 ) ) ;
#21308=VECTOR ( 'NONE', #24110, 1000.000000000000000 ) ;
#21310=FACE_OUTER_BOUND ( 'NONE', #23575, .T. ) ;
#21318=VERTEX_POINT ( 'NONE', #17724 ) ;
#21334=EDGE_CURVE ( 'NONE', #20889, #17789, #22209, .T. ) ;
#21352=LINE ( 'NONE', #1887, #17683 ) ;
#21353=ADVANCED_FACE ( 'NONE', ( #302 ), #23879, .T. ) ;
#21354=ORIENTED_EDGE ( 'NONE', *, *, #12501, .T. ) ;
#21359=AXIS2_PLACEMENT_3D ( 'NONE', #16891, #15329, #20760 ) ;
#21373=DIRECTION ( 'NONE',  ( 0.000000000000000000, -1.000000000000000000, 2.999999999999999839E-15 ) ) ;
#21381=VECTOR ( 'NONE', #11139, 1000.000000000000000 ) ;
#21385=EDGE_LOOP ( 'NONE', ( #21176, #15121, #10071, #12465 ) ) ;
#21393=EDGE_CURVE ( 'NONE', #16850, #14470, #2113, .T. ) ;
#21397=DIRECTION ( 'NONE',  ( 0.000000000000000000, -3.965082230804126670E-15, -1.000000000000000000 ) ) ;
#21401=CARTESIAN_POINT ( 'NONE',  ( 37.31606138205700063, 42.19123852234599781, 74.30501292736987295 ) ) ;
#21420=VECTOR ( 'NONE', #22351, 1000.000000000000000 ) ;
#21426=CARTESIAN_POINT ( 'NONE',  ( 44.81606138205700063, 41.44123852234599781, 74.30501292736987295 ) ) ;
#21432=DIRECTION ( 'NONE',  ( 0.000000000000000000, -2.999999999999999839E-15, -1.000000000000000000 ) ) ;
#21435=EDGE_CURVE ( 'NONE', #24927, #821, #2492, .T. ) ;
#21444=PLANE ( 'NONE',  #11408 ) ;
#21459=PLANE ( 'NONE',  #13480 ) ;
#21467=LINE ( 'NONE', #20966, #12013 ) ;
#21491=VERTEX_POINT ( 'NONE', #18476 ) ;
#21497=PLANE ( 'NONE',  #14206 ) ;
#21498=LINE ( 'NONE', #17381, #9245 ) ;
#21500=ORIENTED_EDGE ( 'NONE', *, *, #18785, .T. ) ;
#21501=CIRCLE ( 'NONE', #8345, 1.549999999999995826 ) ;
#21505=DIRECTION ( 'NONE',  ( 1.000000000000000000, 0.000000000000000000, 0.000000000000000000 ) ) ;
#21509=AXIS2_PLACEMENT_3D ( 'NONE', #17902, #347, #23800 ) ;
#21510=CARTESIAN_POINT ( 'NONE',  ( 43.06606138205700063, -34.55876147765400219, 75.30501292737011454 ) ) ;
#21514=DIRECTION ( 'NONE',  ( 0.000000000000000000, 4.476705744456288765E-15, 1.000000000000000000 ) ) ;
#21525=PLANE ( 'NONE',  #1635 ) ;
#21527=EDGE_CURVE ( 'NONE', #11368, #6775, #3130, .T. ) ;
#21544=DIRECTION ( 'NONE',  ( 0.000000000000000000, -1.000000000000000000, 2.999999999999999839E-15 ) ) ;
#21545=VECTOR ( 'NONE', #23069, 1000.000000000000000 ) ;
#21563=EDGE_LOOP ( 'NONE', ( #3570, #6124 ) ) ;
#21569=CARTESIAN_POINT ( 'NONE',  ( 32.81606138205700773, 35.95440708241085304, 61.30501292736990138 ) ) ;
#21575=STYLED_ITEM ( 'NONE', ( #7929 ), #21819 ) ;
#21580=DIRECTION ( 'NONE',  ( -1.000000000000000000, -6.938893903907188146E-15, 8.673617379884188314E-16 ) ) ;
#21582=CARTESIAN_POINT ( 'NONE',  ( 35.81606138205700063, -31.05876147765399864, 74.30501292737010033 ) ) ;
#21584=DIRECTION ( 'NONE',  ( -1.000000000000000000, 5.352861011585579840E-16, -1.605858303475673768E-30 ) ) ;
#21588=EDGE_CURVE ( 'NONE', #20176, #22023, #17181, .T. ) ;
#21598=DIRECTION ( 'NONE',  ( 0.000000000000000000, 9.938893903907240838E-15, 1.000000000000000000 ) ) ;
#21599=PLANE ( 'NONE',  #6676 ) ;
#21600=ORIENTED_EDGE ( 'NONE', *, *, #16028, .T. ) ;
#21601=DIRECTION ( 'NONE',  ( 1.000000000000000000, -5.510910596163088391E-31, -1.836970198721029688E-16 ) ) ;
#21605=CARTESIAN_POINT ( 'NONE',  ( 35.81606138205700063, 37.44123852234599781, 74.30501292736988717 ) ) ;
#21608=VERTEX_POINT ( 'NONE', #19738 ) ;
#21620=ORIENTED_EDGE ( 'NONE', *, *, #22789, .T. ) ;
#21624=DIRECTION ( 'NONE',  ( 0.000000000000000000, -1.000000000000000000, 2.999999999999999839E-15 ) ) ;
#21633=LINE ( 'NONE', #7125, #549 ) ;
#21640=DIRECTION ( 'NONE',  ( 0.000000000000000000, 1.000000000000000000, 0.000000000000000000 ) ) ;
#21648=ORIENTED_EDGE ( 'NONE', *, *, #23324, .F. ) ;
#21657=CARTESIAN_POINT ( 'NONE',  ( 32.81606138205700773, 18.19123852234599426, 73.05501292736995822 ) ) ;
#21667=EDGE_CURVE ( 'NONE', #15432, #8317, #2212, .T. ) ;
#21673=VECTOR ( 'NONE', #13463, 1000.000000000000000 ) ;
#21682=EDGE_LOOP ( 'NONE', ( #342, #7181, #11918, #19748 ) ) ;
#21684=FACE_OUTER_BOUND ( 'NONE', #22633, .T. ) ;
#21691=VECTOR ( 'NONE', #11110, 1000.000000000000000 ) ;
#21696=CARTESIAN_POINT ( 'NONE',  ( 31.81606138205700418, -34.55876147765400930, 73.30501292737011454 ) ) ;
#21699=DIRECTION ( 'NONE',  ( 0.000000000000000000, 1.000000000000000000, -2.999999999999999839E-15 ) ) ;
#21700=ORIENTED_EDGE ( 'NONE', *, *, #2300, .F. ) ;
#21701=CARTESIAN_POINT ( 'NONE',  ( 37.31606138205700063, 43.19123852234599781, 74.30501292736987295 ) ) ;
#21703=VERTEX_POINT ( 'NONE', #10335 ) ;
#21716=VECTOR ( 'NONE', #13348, 1000.000000000000000 ) ;
#21718=VERTEX_POINT ( 'NONE', #23844 ) ;
#21722=ORIENTED_EDGE ( 'NONE', *, *, #20749, .T. ) ;
#21724=CARTESIAN_POINT ( 'NONE',  ( 33.56606138205700773, 42.19123852234599781, 75.30501292736987295 ) ) ;
#21726=LINE ( 'NONE', #3950, #14888 ) ;
#21734=LINE ( 'NONE', #14260, #20909 ) ;
#21747=ORIENTED_EDGE ( 'NONE', *, *, #3317, .T. ) ;
#21754=EDGE_CURVE ( 'NONE', #9537, #4816, #22049, .T. ) ;
#21756=PLANE ( 'NONE',  #11056 ) ;
#21759=CARTESIAN_POINT ( 'NONE',  ( 43.81606138205700063, 39.55420052130484265, 58.58767820587064534 ) ) ;
#21768=ORIENTED_EDGE ( 'NONE', *, *, #5010, .F. ) ;
#21773=VERTEX_POINT ( 'NONE', #1033 ) ;
#21779=CARTESIAN_POINT ( 'NONE',  ( 44.81606138205700063, 1.441238522345976714, 67.80501292737001506 ) ) ;
#21781=CIRCLE ( 'NONE', #7812, 4.000000000000000000 ) ;
#21800=EDGE_CURVE ( 'NONE', #3791, #17124, #270, .T. ) ;
#21815=VECTOR ( 'NONE', #14727, 1000.000000000000000 ) ;
#21819=ADVANCED_BREP_SHAPE_REPRESENTATION ( '', ( #8398, #2000 ), #6773 ) ;
#21824=FILL_AREA_STYLE_COLOUR ( '', #20766 ) ;
#21825=CARTESIAN_POINT ( 'NONE',  ( 44.81606138205700063, 18.19123852234598715, 71.05501292736995822 ) ) ;
#21837=ORIENTED_EDGE ( 'NONE', *, *, #1540, .F. ) ;
#21838=ORIENTED_EDGE ( 'NONE', *, *, #8085, .T. ) ;
#21849=ADVANCED_FACE ( 'NONE', ( #22178 ), #4662, .F. ) ;
#21852=CARTESIAN_POINT ( 'NONE',  ( 40.81606138205700773, -31.05876147765399864, 75.30501292737010033 ) ) ;
#21853=DIRECTION ( 'NONE',  ( -8.552847072295029957E-47, 1.000000000000000000, -2.999999999999999839E-15 ) ) ;
#21863=DIRECTION ( 'NONE',  ( 0.000000000000000000, 6.938893903907222067E-15, -1.000000000000000000 ) ) ;
#21872=DIRECTION ( 'NONE',  ( 0.000000000000000000, -1.000000000000000000, 3.129456975819164530E-15 ) ) ;
#21880=LINE ( 'NONE', #19684, #16118 ) ;
#21887=VECTOR ( 'NONE', #9511, 1000.000000000000000 ) ;
#21898=ORIENTED_EDGE ( 'NONE', *, *, #2098, .F. ) ;
#21901=PRODUCT_DEFINITION ( 'UNKNOWN', '', #21170, #4385 ) ;
#21906=FACE_OUTER_BOUND ( 'NONE', #12379, .T. ) ;
#21911=FACE_OUTER_BOUND ( 'NONE', #16366, .T. ) ;
#21917=DIRECTION ( 'NONE',  ( 0.000000000000000000, -3.965082230804126670E-15, -1.000000000000000000 ) ) ;
#21918=AXIS2_PLACEMENT_3D ( 'NONE', #23763, #6627, #16409 ) ;
#21920=VECTOR ( 'NONE', #2359, 1000.000000000000000 ) ;
#21937=ORIENTED_EDGE ( 'NONE', *, *, #23909, .T. ) ;
#21943=CARTESIAN_POINT ( 'NONE',  ( 42.06606138205700063, 41.44123852234599781, 74.30501292736987295 ) ) ;
#21946=CARTESIAN_POINT ( 'NONE',  ( 33.56606138205700773, 42.19123852234601202, 79.18605660143489899 ) ) ;
#21960=DIRECTION ( 'NONE',  ( -4.256992727861094749E-32, 1.000000000000000000, -3.115648231731786715E-15 ) ) ;
#21962=AXIS2_PLACEMENT_3D ( 'NONE', #3976, #12589, #10517 ) ;
#21971=ORIENTED_EDGE ( 'NONE', *, *, #10975, .F. ) ;
#21974=CYLINDRICAL_SURFACE ( 'NONE', #5412, 0.7500000000000006661 ) ;
#21978=CARTESIAN_POINT ( 'NONE',  ( 44.81606138205700063, 41.44123852234596939, 66.30501292736988717 ) ) ;
#21979=EDGE_CURVE ( 'NONE', #5370, #6126, #7709, .T. ) ;
#21980=DIRECTION ( 'NONE',  ( 0.000000000000000000, -2.999999999999999839E-15, -1.000000000000000000 ) ) ;
#21981=ORIENTED_EDGE ( 'NONE', *, *, #14272, .F. ) ;
#21989=FACE_OUTER_BOUND ( 'NONE', #21385, .T. ) ;
#21990=FACE_BOUND ( 'NONE', #25233, .T. ) ;
#21996=EDGE_CURVE ( 'NONE', #15888, #8849, #18698, .T. ) ;
#22005=EDGE_CURVE ( 'NONE', #1363, #4055, #5178, .T. ) ;
#22023=VERTEX_POINT ( 'NONE', #16894 ) ;
#22041=CARTESIAN_POINT ( 'NONE',  ( 31.81606138205700418, 38.19123852234599070, 72.05501292736988717 ) ) ;
#22049=LINE ( 'NONE', #12029, #24937 ) ;
#22055=DIRECTION ( 'NONE',  ( 0.000000000000000000, 0.000000000000000000, 1.000000000000000000 ) ) ;
#22062=CARTESIAN_POINT ( 'NONE',  ( 40.31606138205700773, -31.05876147765400574, 73.55501292737010033 ) ) ;
#22066=EDGE_CURVE ( 'NONE', #23642, #17124, #10171, .T. ) ;
#22068=ADVANCED_FACE ( 'NONE', ( #357 ), #12373, .F. ) ;
#22080=ORIENTED_EDGE ( 'NONE', *, *, #24203, .T. ) ;
#22086=CYLINDRICAL_SURFACE ( 'NONE', #10816, 1.000000000000000888 ) ;
#22091=VERTEX_POINT ( 'NONE', #23936 ) ;
#22097=AXIS2_PLACEMENT_3D ( 'NONE', #9070, #19103, #1441 ) ;
#22099=AXIS2_PLACEMENT_3D ( 'NONE', #20271, #6110, #13969 ) ;
#22100=AXIS2_PLACEMENT_3D ( 'NONE', #6840, #14695, #22559 ) ;
#22109=PLANE ( 'NONE',  #12046 ) ;
#22113=CARTESIAN_POINT ( 'NONE',  ( 36.31606138205700063, -30.30876147765401996, 69.30501292737010033 ) ) ;
#22120=ORIENTED_EDGE ( 'NONE', *, *, #22816, .F. ) ;
#22126=CARTESIAN_POINT ( 'NONE',  ( 39.31606138205700063, 43.19123852234599781, 74.30501292736987295 ) ) ;
#22130=VECTOR ( 'NONE', #16517, 1000.000000000000000 ) ;
#22134=EDGE_CURVE ( 'NONE', #4343, #19498, #13909, .T. ) ;
#22144=ORIENTED_EDGE ( 'NONE', *, *, #23041, .T. ) ;
#22145=ORIENTED_EDGE ( 'NONE', *, *, #22134, .T. ) ;
#22153=CARTESIAN_POINT ( 'NONE',  ( 37.31606138205700063, 42.19123852234596939, 66.30501292736988717 ) ) ;
#22154=LINE ( 'NONE', #20227, #7985 ) ;
#22159=CARTESIAN_POINT ( 'NONE',  ( 36.31606138205700063, 42.19123852234599781, 75.30501292736987295 ) ) ;
#22176=EDGE_CURVE ( 'NONE', #2388, #6126, #23688, .T. ) ;
#22178=FACE_OUTER_BOUND ( 'NONE', #4077, .T. ) ;
#22199=CARTESIAN_POINT ( 'NONE',  ( 31.81606138205700418, 41.44123852234595518, 61.30501292736988006 ) ) ;
#22203=PLANE ( 'NONE',  #518 ) ;
#22205=DIRECTION ( 'NONE',  ( 0.000000000000000000, -1.000000000000000000, 2.999999999999999839E-15 ) ) ;
#22208=VECTOR ( 'NONE', #20537, 1000.000000000000000 ) ;
#22209=LINE ( 'NONE', #17977, #5755 ) ;
#22210=ORIENTED_EDGE ( 'NONE', *, *, #13250, .T. ) ;
#22212=ORIENTED_EDGE ( 'NONE', *, *, #21334, .T. ) ;
#22215=DIRECTION ( 'NONE',  ( 0.000000000000000000, 1.000000000000000000, 0.000000000000000000 ) ) ;
#22216=EDGE_CURVE ( 'NONE', #12889, #4199, #18413, .T. ) ;
#22217=VECTOR ( 'NONE', #179, 1000.000000000000000 ) ;
#22224=CARTESIAN_POINT ( 'NONE',  ( 34.56606138205700773, 42.19123852234599781, 75.30501292736987295 ) ) ;
#22243=DIRECTION ( 'NONE',  ( 1.000000000000000000, -5.352861011585579840E-16, 1.605858303475673768E-30 ) ) ;
#22252=ORIENTED_EDGE ( 'NONE', *, *, #6170, .T. ) ;
#22257=VECTOR ( 'NONE', #14108, 1000.000000000000000 ) ;
#22258=DIRECTION ( 'NONE',  ( 0.000000000000000000, 1.000000000000000000, -2.999999999999999839E-15 ) ) ;
#22262=ADVANCED_FACE ( 'NONE', ( #8625 ), #16989, .T. ) ;
#22281=DIRECTION ( 'NONE',  ( -3.491481338843135327E-15, 1.000000000000000000, -2.999999999999999050E-15 ) ) ;
#22283=AXIS2_PLACEMENT_3D ( 'NONE', #15692, #21624, #222 ) ;
#22287=DIRECTION ( 'NONE',  ( 3.717264591378870232E-16, 3.130104260698260371E-15, 1.000000000000000000 ) ) ;
#22289=VECTOR ( 'NONE', #719, 1000.000000000000000 ) ;
#22309=CARTESIAN_POINT ( 'NONE',  ( 36.31606138205700063, 37.94123852234599781, 75.30501292736988717 ) ) ;
#22311=CARTESIAN_POINT ( 'NONE',  ( 35.81606138205700063, -31.05876147765399864, 75.30501292737010033 ) ) ;
#22313=EDGE_CURVE ( 'NONE', #15455, #23735, #24556, .T. ) ;
#22316=ORIENTED_EDGE ( 'NONE', *, *, #14678, .T. ) ;
#22320=CYLINDRICAL_SURFACE ( 'NONE', #12839, 1.000000000000000888 ) ;
#22322=CARTESIAN_POINT ( 'NONE',  ( 38.31606138205700063, -29.30876147765400930, 71.30501292737010033 ) ) ;
#22324=CARTESIAN_POINT ( 'NONE',  ( 33.56606138205700773, 41.44123852234599070, 73.55501292736987295 ) ) ;
#22327=VERTEX_POINT ( 'NONE', #6938 ) ;
#22340=AXIS2_PLACEMENT_3D ( 'NONE', #19122, #23345, #23098 ) ;
#22343=ORIENTED_EDGE ( 'NONE', *, *, #10182, .F. ) ;
#22345=VECTOR ( 'NONE', #1187, 1000.000000000000000 ) ;
#22346=CYLINDRICAL_SURFACE ( 'NONE', #11297, 0.5000000000000004441 ) ;
#22350=ORIENTED_EDGE ( 'NONE', *, *, #24060, .T. ) ;
#22351=DIRECTION ( 'NONE',  ( 0.000000000000000000, 1.000000000000000000, -2.999999999999999839E-15 ) ) ;
#22353=CARTESIAN_POINT ( 'NONE',  ( 32.81606138205700773, 41.44123852234595518, 61.30501292736988006 ) ) ;
#22358=CARTESIAN_POINT ( 'NONE',  ( 40.81606138205700773, 41.44123852234599781, 75.30501292736988717 ) ) ;
#22361=ORIENTED_EDGE ( 'NONE', *, *, #15238, .F. ) ;
#22368=DIRECTION ( 'NONE',  ( 0.000000000000000000, 1.000000000000000000, -2.999999999999999839E-15 ) ) ;
#22370=AXIS2_PLACEMENT_3D ( 'NONE', #12388, #9943, #6200 ) ;
#22371=DIRECTION ( 'NONE',  ( 1.000000000000000000, 0.000000000000000000, 0.000000000000000000 ) ) ;
#22373=AXIS2_PLACEMENT_3D ( 'NONE', #11991, #18976, #11124 ) ;
#22375=ORIENTED_EDGE ( 'NONE', *, *, #20629, .F. ) ;
#22381=EDGE_LOOP ( 'NONE', ( #21768, #3820, #22343, #958 ) ) ;
#22388=CIRCLE ( 'NONE', #22788, 0.7500000000000006661 ) ;
#22391=DIRECTION ( 'NONE',  ( 1.734723475976805122E-15, 2.999999999999999839E-15, 1.000000000000000000 ) ) ;
#22393=ADVANCED_FACE ( 'NONE', ( #15044 ), #5263, .T. ) ;
#22397=DIRECTION ( 'NONE',  ( 0.000000000000000000, 1.000000000000000000, -2.999999999999999839E-15 ) ) ;
#22415=VECTOR ( 'NONE', #13805, 1000.000000000000000 ) ;
#22422=CARTESIAN_POINT ( 'NONE',  ( 35.31606138205687273, 43.19123852234596939, 65.30501292736988717 ) ) ;
#22427=ORIENTED_EDGE ( 'NONE', *, *, #14937, .T. ) ;
#22433=VERTEX_POINT ( 'NONE', #13631 ) ;
#22439=CARTESIAN_POINT ( 'NONE',  ( 43.81606138205700063, 41.44123852234595518, 61.30501292736988006 ) ) ;
#22447=CARTESIAN_POINT ( 'NONE',  ( 44.81606138205700063, -36.10876147765401356, 70.30501292737011454 ) ) ;
#22451=DIRECTION ( 'NONE',  ( 1.000000000000000000, 0.000000000000000000, 0.000000000000000000 ) ) ;
#22462=ORIENTED_EDGE ( 'NONE', *, *, #23401, .F. ) ;
#22463=ADVANCED_FACE ( 'NONE', ( #24935 ), #7707, .F. ) ;
#22466=ORIENTED_EDGE ( 'NONE', *, *, #13372, .F. ) ;
#22475=DIRECTION ( 'NONE',  ( 3.717264591378870232E-16, 2.999999999999999839E-15, 1.000000000000000000 ) ) ;
#22480=FACE_OUTER_BOUND ( 'NONE', #21682, .T. ) ;
#22485=CARTESIAN_POINT ( 'NONE',  ( 33.56606138205700773, 43.19123852234599781, 74.30501292736987295 ) ) ;
#22493=CARTESIAN_POINT ( 'NONE',  ( 43.81606138205700063, 18.19123852234599426, 73.05501292736995822 ) ) ;
#22497=ORIENTED_EDGE ( 'NONE', *, *, #3341, .T. ) ;
#22507=DIRECTION ( 'NONE',  ( 0.000000000000000000, 1.000000000000000000, -2.999999999999999839E-15 ) ) ;
#22511=EDGE_CURVE ( 'NONE', #7904, #19498, #25065, .T. ) ;
#22514=CARTESIAN_POINT ( 'NONE',  ( 44.81606138205700063, 38.19123852234599070, 72.05501292736988717 ) ) ;
#22515=CARTESIAN_POINT ( 'NONE',  ( 33.56606138205700773, 41.44123852234599781, 74.30501292736987295 ) ) ;
#22525=LINE ( 'NONE', #16862, #18542 ) ;
#22527=ORIENTED_EDGE ( 'NONE', *, *, #11171, .T. ) ;
#22531=AXIS2_PLACEMENT_3D ( 'NONE', #8347, #596, #20061 ) ;
#22535=VECTOR ( 'NONE', #16182, 1000.000000000000000 ) ;
#22537=DIRECTION ( 'NONE',  ( 1.000000000000000000, 0.000000000000000000, 0.000000000000000000 ) ) ;
#22539=CARTESIAN_POINT ( 'NONE',  ( 32.81606138205700773, 35.44123852234597649, 67.80501292736990138 ) ) ;
#22550=EDGE_CURVE ( 'NONE', #13391, #2309, #21352, .T. ) ;
#22557=ORIENTED_EDGE ( 'NONE', *, *, #6948, .F. ) ;
#22559=DIRECTION ( 'NONE',  ( 0.000000000000000000, 6.938893903907222067E-15, -1.000000000000000000 ) ) ;
#22563=VERTEX_POINT ( 'NONE', #22113 ) ;
#22574=FACE_BOUND ( 'NONE', #8225, .T. ) ;
#22576=VECTOR ( 'NONE', #17650, 1000.000000000000000 ) ;
#22583=LINE ( 'NONE', #16786, #17836 ) ;
#22586=CARTESIAN_POINT ( 'NONE',  ( 44.81606138205700063, 28.69846577177642288, 66.12638289304319983 ) ) ;
#22601=EDGE_LOOP ( 'NONE', ( #19149, #18357, #5381, #2223 ) ) ;
#22611=ORIENTED_EDGE ( 'NONE', *, *, #22948, .F. ) ;
#22612=VECTOR ( 'NONE', #23151, 1000.000000000000000 ) ;
#22622=CARTESIAN_POINT ( 'NONE',  ( 31.81606138205700418, 35.44123852234597649, 68.80501292736990138 ) ) ;
#22624=DIRECTION ( 'NONE',  ( 0.000000000000000000, 1.000000000000000000, 0.000000000000000000 ) ) ;
#22627=CARTESIAN_POINT ( 'NONE',  ( 40.31606138205700773, -31.05876147765399864, 75.30501292737010033 ) ) ;
#22628=LINE ( 'NONE', #5372, #18504 ) ;
#22633=EDGE_LOOP ( 'NONE', ( #25210, #4027, #14628, #13598 ) ) ;
#22639=AXIS2_PLACEMENT_3D ( 'NONE', #12006, #2434, #16341 ) ;
#22648=DIRECTION ( 'NONE',  ( 1.000000000000000000, -3.083952846180990083E-15, 9.251858538542970050E-30 ) ) ;
#22655=DIRECTION ( 'NONE',  ( -1.000000000000000000, 5.204170427930413997E-31, 1.734723475976804876E-16 ) ) ;
#22656=ORIENTED_EDGE ( 'NONE', *, *, #13903, .T. ) ;
#22680=DIRECTION ( 'NONE',  ( 1.000000000000000000, 1.115287202090205222E-30, -1.734723475976805122E-15 ) ) ;
#22684=CARTESIAN_POINT ( 'NONE',  ( 36.31606138205700063, 42.19123852234596939, 65.30501292736988717 ) ) ;
#22686=EDGE_LOOP ( 'NONE', ( #12664, #2365, #13732, #22957, #18512, #18605, #22851, #12771, #12637, #10215, #22210 ) ) ;
#22693=DIRECTION ( 'NONE',  ( -1.000000000000000000, 1.115179377413661005E-30, 3.717264591378870232E-16 ) ) ;
#22701=FACE_OUTER_BOUND ( 'NONE', #23062, .T. ) ;
#22703=CYLINDRICAL_SURFACE ( 'NONE', #132, 1.750000000000001554 ) ;
#22707=VECTOR ( 'NONE', #11461, 1000.000000000000000 ) ;
#22709=LINE ( 'NONE', #2859, #11678 ) ;
#22724=ORIENTED_EDGE ( 'NONE', *, *, #12078, .T. ) ;
#22725=EDGE_LOOP ( 'NONE', ( #19967, #1298, #16573, #2680 ) ) ;
#22732=AXIS2_PLACEMENT_3D ( 'NONE', #5505, #1107, #18902 ) ;
#22738=AXIS2_PLACEMENT_3D ( 'NONE', #17522, #21373, #1781 ) ;
#22747=CARTESIAN_POINT ( 'NONE',  ( 33.56606138205700773, -38.55876147765401640, 71.30501292737012875 ) ) ;
#22773=EDGE_CURVE ( 'NONE', #10464, #9429, #8215, .T. ) ;
#22775=VECTOR ( 'NONE', #15573, 1000.000000000000000 ) ;
#22776=DIRECTION ( 'NONE',  ( 1.000000000000000000, 0.000000000000000000, 0.000000000000000000 ) ) ;
#22780=ORIENTED_EDGE ( 'NONE', *, *, #796, .F. ) ;
#22787=CIRCLE ( 'NONE', #18281, 0.9999999999999940048 ) ;
#22788=AXIS2_PLACEMENT_3D ( 'NONE', #15005, #25023, #19002 ) ;
#22789=EDGE_CURVE ( 'NONE', #6972, #5864, #18379, .T. ) ;
#22793=VERTEX_POINT ( 'NONE', #22622 ) ;
#22794=DIRECTION ( 'NONE',  ( 0.000000000000000000, -1.000000000000000000, 2.999999999999999839E-15 ) ) ;
#22812=DIRECTION ( 'NONE',  ( 0.000000000000000000, 1.000000000000000000, 0.000000000000000000 ) ) ;
#22816=EDGE_CURVE ( 'NONE', #23642, #18207, #21781, .T. ) ;
#22822=AXIS2_PLACEMENT_3D ( 'NONE', #12551, #18208, #20387 ) ;
#22824=DIRECTION ( 'NONE',  ( -3.717264591378870232E-16, -2.999999999999999839E-15, -1.000000000000000000 ) ) ;
#22825=VERTEX_POINT ( 'NONE', #22493 ) ;
#22826=DIRECTION ( 'NONE',  ( 0.000000000000000000, 1.000000000000000000, -2.913263826201159484E-15 ) ) ;
#22833=CARTESIAN_POINT ( 'NONE',  ( 35.31606138205687273, 42.19123852234596939, 65.30501292736988717 ) ) ;
#22836=CARTESIAN_POINT ( 'NONE',  ( 40.31606138205700773, -29.30876147765401640, 69.30501292737010033 ) ) ;
#22842=CARTESIAN_POINT ( 'NONE',  ( 44.81606138205700063, 28.12806996228107081, 65.30501292736992980 ) ) ;
#22849=PLANE ( 'NONE',  #17466 ) ;
#22851=ORIENTED_EDGE ( 'NONE', *, *, #21393, .T. ) ;
#22863=ORIENTED_EDGE ( 'NONE', *, *, #16265, .F. ) ;
#22873=EDGE_CURVE ( 'NONE', #13029, #13874, #11941, .T. ) ;
#22878=DIRECTION ( 'NONE',  ( 0.000000000000000000, 1.163336342344335610E-15, -1.000000000000000000 ) ) ;
#22895=CARTESIAN_POINT ( 'NONE',  ( 38.31606138205700063, 38.69123852234599781, 75.30501292737004349 ) ) ;
#22898=DIRECTION ( 'NONE',  ( 1.000000000000000000, -1.115179377413661005E-30, -3.717264591378870232E-16 ) ) ;
#22901=VERTEX_POINT ( 'NONE', #6787 ) ;
#22924=DIRECTION ( 'NONE',  ( 5.664403186863039509E-16, 3.000000000000000628E-15, 1.000000000000000000 ) ) ;
#22933=VECTOR ( 'NONE', #9350, 1000.000000000000000 ) ;
#22943=EDGE_CURVE ( 'NONE', #3712, #17085, #10780, .T. ) ;
#22945=CARTESIAN_POINT ( 'NONE',  ( 44.81606138205700063, 35.44123852234597649, 68.80501292736990138 ) ) ;
#22946=FACE_OUTER_BOUND ( 'NONE', #18587, .T. ) ;
#22948=EDGE_CURVE ( 'NONE', #13145, #24731, #7035, .T. ) ;
#22950=EDGE_CURVE ( 'NONE', #9537, #821, #12976, .T. ) ;
#22957=ORIENTED_EDGE ( 'NONE', *, *, #5010, .T. ) ;
#22979=DIRECTION ( 'NONE',  ( 0.000000000000000000, 1.000000000000000000, 0.000000000000000000 ) ) ;
#22984=DIRECTION ( 'NONE',  ( 1.000000000000000000, 0.000000000000000000, 0.000000000000000000 ) ) ;
#22986=ORIENTED_EDGE ( 'NONE', *, *, #10810, .T. ) ;
#22988=CARTESIAN_POINT ( 'NONE',  ( 35.81606138205700063, 37.44123852234599781, 75.30501292736990138 ) ) ;
#22992=DIRECTION ( 'NONE',  ( 0.000000000000000000, 3.469446951953611033E-15, 1.000000000000000000 ) ) ;
#22993=VECTOR ( 'NONE', #6376, 1000.000000000000000 ) ;
#22997=DIRECTION ( 'NONE',  ( 0.000000000000000000, -1.000000000000000000, 0.000000000000000000 ) ) ;
#23005=CARTESIAN_POINT ( 'NONE',  ( 36.31606138205700063, 39.69123852234599070, 73.55501292736988717 ) ) ;
#23009=ORIENTED_EDGE ( 'NONE', *, *, #16629, .T. ) ;
#23016=VECTOR ( 'NONE', #12697, 1000.000000000000000 ) ;
#23021=VECTOR ( 'NONE', #837, 1000.000000000000000 ) ;
#23026=ADVANCED_FACE ( 'NONE', ( #23118 ), #3293, .T. ) ;
#23028=LINE ( 'NONE', #18663, #22612 ) ;
#23034=CIRCLE ( 'NONE', #12777, 1.000000000000000888 ) ;
#23038=VERTEX_POINT ( 'NONE', #15402 ) ;
#23040=DIRECTION ( 'NONE',  ( 0.000000000000000000, -1.000000000000000000, 2.999999999999999839E-15 ) ) ;
#23041=EDGE_CURVE ( 'NONE', #5522, #10597, #15650, .T. ) ;
#23053=ORIENTED_EDGE ( 'NONE', *, *, #15120, .F. ) ;
#23057=ORIENTED_EDGE ( 'NONE', *, *, #16568, .F. ) ;
#23060=PRODUCT_DEFINITION_SHAPE ( 'NONE', 'NONE',  #21901 ) ;
#23062=EDGE_LOOP ( 'NONE', ( #11004, #1952, #10128, #9876 ) ) ;
#23069=DIRECTION ( 'NONE',  ( 0.000000000000000000, -2.999999999999999839E-15, -1.000000000000000000 ) ) ;
#23076=DIRECTION ( 'NONE',  ( 1.000000000000000000, 0.000000000000000000, 0.000000000000000000 ) ) ;
#23097=CARTESIAN_POINT ( 'NONE',  ( 42.06606138205700063, 42.19123852234599781, 75.30501292736987295 ) ) ;
#23098=DIRECTION ( 'NONE',  ( 0.000000000000000000, -3.469446951953611033E-15, 1.000000000000000000 ) ) ;
#23101=ORIENTED_EDGE ( 'NONE', *, *, #12417, .F. ) ;
#23104=CARTESIAN_POINT ( 'NONE',  ( 38.31606138205700063, 42.51966564709218943, 72.30501292737018559 ) ) ;
#23116=ORIENTED_EDGE ( 'NONE', *, *, #18849, .T. ) ;
#23118=FACE_OUTER_BOUND ( 'NONE', #21259, .T. ) ;
#23132=VECTOR ( 'NONE', #17992, 1000.000000000000000 ) ;
#23133=DIRECTION ( 'NONE',  ( 0.000000000000000000, -2.999999999999999839E-15, -1.000000000000000000 ) ) ;
#23140=EDGE_LOOP ( 'NONE', ( #19971, #7557, #12853, #22611 ) ) ;
#23151=DIRECTION ( 'NONE',  ( -1.000000000000000000, 1.115179377413661005E-30, 3.717264591378870232E-16 ) ) ;
#23152=AXIS2_PLACEMENT_3D ( 'NONE', #16297, #12208, #20052 ) ;
#23155=ORIENTED_EDGE ( 'NONE', *, *, #141, .T. ) ;
#23163=VECTOR ( 'NONE', #15217, 1000.000000000000000 ) ;
#23171=VECTOR ( 'NONE', #6860, 1000.000000000000000 ) ;
#23174=DIRECTION ( 'NONE',  ( -1.836970198721029688E-16, -2.999999999999999839E-15, -1.000000000000000000 ) ) ;
#23182=VECTOR ( 'NONE', #23040, 1000.000000000000000 ) ;
#23189=ORIENTED_EDGE ( 'NONE', *, *, #15709, .T. ) ;
#23195=DIRECTION ( 'NONE',  ( 0.000000000000000000, 1.000000000000000000, -6.938893903907222067E-15 ) ) ;
#23213=CIRCLE ( 'NONE', #12143, 1.000000000000000888 ) ;
#23224=ORIENTED_EDGE ( 'NONE', *, *, #9177, .F. ) ;
#23225=ORIENTED_EDGE ( 'NONE', *, *, #23733, .T. ) ;
#23229=DIRECTION ( 'NONE',  ( -9.027796614315171564E-31, -1.000000000000000000, -1.163336342344335610E-15 ) ) ;
#23231=ADVANCED_FACE ( 'NONE', ( #23498 ), #4441, .F. ) ;
#23232=DIRECTION ( 'NONE',  ( 9.027796614315171564E-31, 1.000000000000000000, 4.694469519536151390E-16 ) ) ;
#23234=CYLINDRICAL_SURFACE ( 'NONE', #8143, 1.750000000000001554 ) ;
#23235=EDGE_LOOP ( 'NONE', ( #12487, #1066, #7827, #16552 ) ) ;
#23260=CARTESIAN_POINT ( 'NONE',  ( 31.81606138205700418, -34.55876147765400930, 73.55501292737011454 ) ) ;
#23262=ORIENTED_EDGE ( 'NONE', *, *, #20629, .T. ) ;
#23269=EDGE_CURVE ( 'NONE', #25152, #1727, #24000, .T. ) ;
#23271=EDGE_CURVE ( 'NONE', #14131, #21718, #14406, .T. ) ;
#23275=CARTESIAN_POINT ( 'NONE',  ( 32.81606138205700773, -34.55876147765401640, 70.30501292737011454 ) ) ;
#23288=ORIENTED_EDGE ( 'NONE', *, *, #21996, .T. ) ;
#23289=DIRECTION ( 'NONE',  ( 0.000000000000000000, 1.000000000000000000, -2.999999999999999839E-15 ) ) ;
#23290=CARTESIAN_POINT ( 'NONE',  ( 43.81606138205700063, 28.12806996228107081, 65.30501292736992980 ) ) ;
#23293=CARTESIAN_POINT ( 'NONE',  ( 40.31606138205700773, 37.94123852234599781, 75.30501292736988717 ) ) ;
#23310=EDGE_LOOP ( 'NONE', ( #17035, #9843, #13642, #14689, #15340, #4446 ) ) ;
#23315=VECTOR ( 'NONE', #14236, 1000.000000000000000 ) ;
#23318=LINE ( 'NONE', #9439, #197 ) ;
#23319=CARTESIAN_POINT ( 'NONE',  ( 37.31606138205700063, 43.19123852234595518, 61.30501292736988006 ) ) ;
#23323=CYLINDRICAL_SURFACE ( 'NONE', #17504, 1.000000000000000888 ) ;
#23324=EDGE_CURVE ( 'NONE', #20889, #64, #14479, .T. ) ;
#23327=DIRECTION ( 'NONE',  ( 0.000000000000000000, -1.000000000000000000, 2.999999999999999839E-15 ) ) ;
#23329=AXIS2_PLACEMENT_3D ( 'NONE', #25243, #13420, #15593 ) ;
#23345=DIRECTION ( 'NONE',  ( -9.027796614315171564E-31, -1.000000000000000000, -3.938893903907230117E-15 ) ) ;
#23380=ORIENTED_EDGE ( 'NONE', *, *, #16339, .F. ) ;
#23383=DIRECTION ( 'NONE',  ( 1.000000000000000000, 0.000000000000000000, 0.000000000000000000 ) ) ;
#23390=ORIENTED_EDGE ( 'NONE', *, *, #16028, .F. ) ;
#23391=CIRCLE ( 'NONE', #16403, 1.000000000000000888 ) ;
#23399=VECTOR ( 'NONE', #13031, 1000.000000000000000 ) ;
#23401=EDGE_CURVE ( 'NONE', #19565, #9905, #19080, .T. ) ;
#23402=ORIENTED_EDGE ( 'NONE', *, *, #9873, .F. ) ;
#23411=AXIS2_PLACEMENT_3D ( 'NONE', #24465, #14323, #12276 ) ;
#23413=CARTESIAN_POINT ( 'NONE',  ( 37.31606138205700063, 43.19123852234596939, 66.30501292736988717 ) ) ;
#23419=PLANE ( 'NONE',  #3462 ) ;
#23441=EDGE_LOOP ( 'NONE', ( #18078, #7066, #9661, #8474, #5999 ) ) ;
#23451=DIRECTION ( 'NONE',  ( 0.000000000000000000, -1.000000000000000000, 2.999999999999999839E-15 ) ) ;
#23452=DIRECTION ( 'NONE',  ( 0.000000000000000000, -1.000000000000000000, 2.999999999999999839E-15 ) ) ;
#23464=DIRECTION ( 'NONE',  ( -1.000000000000000000, 0.000000000000000000, 0.000000000000000000 ) ) ;
#23481=CARTESIAN_POINT ( 'NONE',  ( 33.56606138205700773, 42.19123852234595518, 61.30501292736988006 ) ) ;
#23488=ORIENTED_EDGE ( 'NONE', *, *, #12078, .F. ) ;
#23494=DIRECTION ( 'NONE',  ( -1.000000000000000000, 1.301042606982604506E-30, 4.336808689942015271E-16 ) ) ;
#23498=FACE_OUTER_BOUND ( 'NONE', #3654, .T. ) ;
#23505=ORIENTED_EDGE ( 'NONE', *, *, #14826, .T. ) ;
#23511=DIRECTION ( 'NONE',  ( 1.000000000000000000, -5.510910596163088391E-31, -1.836970198721029688E-16 ) ) ;
#23513=EDGE_LOOP ( 'NONE', ( #2885, #25133, #20922, #1227 ) ) ;
#23514=DIRECTION ( 'NONE',  ( -9.027796614315171564E-31, -1.000000000000000000, -1.163336342344335610E-15 ) ) ;
#23519=CARTESIAN_POINT ( 'NONE',  ( 32.81606138205700773, 41.44123852234595518, 61.30501292736988006 ) ) ;
#23521=EDGE_LOOP ( 'NONE', ( #18788, #10626, #19249, #2688 ) ) ;
#23531=DIRECTION ( 'NONE',  ( 1.000000000000000000, 3.491481338843134144E-15, -3.540251991789504463E-16 ) ) ;
#23566=AXIS2_PLACEMENT_3D ( 'NONE', #3397, #7780, #11654 ) ;
#23568=ORIENTED_EDGE ( 'NONE', *, *, #1761, .T. ) ;
#23575=EDGE_LOOP ( 'NONE', ( #15660, #13861, #15434, #18750 ) ) ;
#23578=CARTESIAN_POINT ( 'NONE',  ( 36.31606138205700063, -29.30876147765401640, 69.30501292737010033 ) ) ;
#23580=AXIS2_PLACEMENT_3D ( 'NONE', #24486, #22451, #20395 ) ;
#23601=ADVANCED_FACE ( 'NONE', ( #7736 ), #3992, .F. ) ;
#23616=ORIENTED_EDGE ( 'NONE', *, *, #5103, .T. ) ;
#23627=ORIENTED_EDGE ( 'NONE', *, *, #66, .T. ) ;
#23631=DIRECTION ( 'NONE',  ( 1.000000000000000000, 0.000000000000000000, 0.000000000000000000 ) ) ;
#23633=LINE ( 'NONE', #10621, #22345 ) ;
#23635=LINE ( 'NONE', #9862, #2011 ) ;
#23636=CARTESIAN_POINT ( 'NONE',  ( 32.81606138205700773, 32.99511671078946762, 63.14259751872857152 ) ) ;
#23642=VERTEX_POINT ( 'NONE', #19446 ) ;
#23647=ADVANCED_FACE ( 'NONE', ( #19578 ), #118, .F. ) ;
#23653=CARTESIAN_POINT ( 'NONE',  ( 43.06606138205700063, 41.44123852234595518, 61.30501292736988006 ) ) ;
#23658=CARTESIAN_POINT ( 'NONE',  ( 44.81606138205700063, -24.55876147765401285, 70.30501292737008612 ) ) ;
#23670=CIRCLE ( 'NONE', #11345, 0.7500000000000006661 ) ;
#23674=ORIENTED_EDGE ( 'NONE', *, *, #24985, .F. ) ;
#23679=VERTEX_POINT ( 'NONE', #2428 ) ;
#23682=SURFACE_STYLE_FILL_AREA ( #15827 ) ;
#23688=LINE ( 'NONE', #2675, #23806 ) ;
#23693=ORIENTED_EDGE ( 'NONE', *, *, #9470, .F. ) ;
#23704=DIRECTION ( 'NONE',  ( -8.673617379884039170E-17, 1.163336342344335610E-15, -1.000000000000000000 ) ) ;
#23728=ORIENTED_EDGE ( 'NONE', *, *, #18675, .T. ) ;
#23733=EDGE_CURVE ( 'NONE', #25254, #9967, #744, .T. ) ;
#23734=VERTEX_POINT ( 'NONE', #2678 ) ;
#23735=VERTEX_POINT ( 'NONE', #8501 ) ;
#23739=CARTESIAN_POINT ( 'NONE',  ( 36.31606138205700063, 37.94123852234599781, 74.30501292736988717 ) ) ;
#23761=ORIENTED_EDGE ( 'NONE', *, *, #16177, .F. ) ;
#23763=CARTESIAN_POINT ( 'NONE',  ( 39.31606138205700063, 43.19123852234595518, 61.30501292736988006 ) ) ;
#23766=AXIS2_PLACEMENT_3D ( 'NONE', #9615, #11158, #24782 ) ;
#23770=CARTESIAN_POINT ( 'NONE',  ( 39.31606138205700063, 42.19123852234599781, 75.30501292736987295 ) ) ;
#23771=CARTESIAN_POINT ( 'NONE',  ( 44.81606138205700063, -34.55876147765401640, 70.30501292737011454 ) ) ;
#23777=CARTESIAN_POINT ( 'NONE',  ( 39.31606138205700063, 43.19123852234599070, 73.55501292736987295 ) ) ;
#23784=FACE_BOUND ( 'NONE', #23441, .T. ) ;
#23788=DIRECTION ( 'NONE',  ( -1.000000000000000000, 0.000000000000000000, 0.000000000000000000 ) ) ;
#23800=DIRECTION ( 'NONE',  ( 0.000000000000000000, -1.000000000000000000, 3.325260651745651169E-15 ) ) ;
#23803=PLANE ( 'NONE',  #93 ) ;
#23804=EDGE_CURVE ( 'NONE', #14470, #20311, #19969, .T. ) ;
#23806=VECTOR ( 'NONE', #6053, 1000.000000000000000 ) ;
#23813=EDGE_LOOP ( 'NONE', ( #16279, #14240, #1681, #4737 ) ) ;
#23816=ORIENTED_EDGE ( 'NONE', *, *, #10810, .F. ) ;
#23819=VECTOR ( 'NONE', #18290, 1000.000000000000000 ) ;
#23830=AXIS2_PLACEMENT_3D ( 'NONE', #10808, #20596, #8629 ) ;
#23833=CARTESIAN_POINT ( 'NONE',  ( 44.81606138205700063, 1.441238522345979600, 68.80501292737000085 ) ) ;
#23844=CARTESIAN_POINT ( 'NONE',  ( 43.81606138205700063, -38.55876147765401640, 70.30501292737012875 ) ) ;
#23849=CARTESIAN_POINT ( 'NONE',  ( 31.81606138205700418, 18.19123852234598715, 71.05501292736995822 ) ) ;
#23856=LINE ( 'NONE', #12422, #6694 ) ;
#23859=DIRECTION ( 'NONE',  ( -1.000000000000000000, 5.204170427930415223E-30, 1.734723475976805122E-15 ) ) ;
#23868=ADVANCED_FACE ( 'NONE', ( #18297 ), #14042, .F. ) ;
#23872=EDGE_CURVE ( 'NONE', #9810, #3466, #17123, .T. ) ;
#23879=PLANE ( 'NONE',  #18921 ) ;
#23885=CARTESIAN_POINT ( 'NONE',  ( 44.81606138205700063, -24.55876147765401996, 67.80501292737008612 ) ) ;
#23892=EDGE_LOOP ( 'NONE', ( #8906, #23288, #14257, #18277 ) ) ;
#23898=DIRECTION ( 'NONE',  ( 0.000000000000000000, -1.000000000000000000, 2.999999999999999839E-15 ) ) ;
#23902=VECTOR ( 'NONE', #13370, 1000.000000000000000 ) ;
#23904=CARTESIAN_POINT ( 'NONE',  ( 33.56606138205700773, 43.19123852234601202, 79.18605660143489899 ) ) ;
#23906=DIRECTION ( 'NONE',  ( -1.000000000000000000, 1.115179377413661005E-30, 3.717264591378870232E-16 ) ) ;
#23909=EDGE_CURVE ( 'NONE', #15432, #1244, #10692, .T. ) ;
#23925=CARTESIAN_POINT ( 'NONE',  ( 41.31606138205687273, 33.19123852234596939, 65.30501292736991559 ) ) ;
#23926=EDGE_CURVE ( 'NONE', #20311, #4444, #10309, .T. ) ;
#23934=VECTOR ( 'NONE', #6698, 1000.000000000000000 ) ;
#23936=CARTESIAN_POINT ( 'NONE',  ( 32.81606138205700773, -36.10876147765401356, 70.30501292737011454 ) ) ;
#23938=ORIENTED_EDGE ( 'NONE', *, *, #10359, .T. ) ;
#23941=EDGE_LOOP ( 'NONE', ( #2343, #23505, #19327, #3798 ) ) ;
#23946=CARTESIAN_POINT ( 'NONE',  ( 44.81606138205700063, -24.55876147765400574, 72.80501292737008612 ) ) ;
#23956=CARTESIAN_POINT ( 'NONE',  ( 41.31606138205687273, 42.19123852234599781, 75.30501292736987295 ) ) ;
#23995=EDGE_CURVE ( 'NONE', #17824, #2309, #24696, .T. ) ;
#24000=LINE ( 'NONE', #9991, #22217 ) ;
#24002=CARTESIAN_POINT ( 'NONE',  ( 33.56606138205700773, 42.19123852234601202, 79.18605660143489899 ) ) ;
#24003=EDGE_LOOP ( 'NONE', ( #6600, #15796, #7578, #20552 ) ) ;
#24011=EDGE_CURVE ( 'NONE', #24485, #21068, #22525, .T. ) ;
#24017=DIRECTION ( 'NONE',  ( 1.000000000000000000, 0.000000000000000000, 0.000000000000000000 ) ) ;
#24029=ORIENTED_EDGE ( 'NONE', *, *, #16846, .T. ) ;
#24031=LINE ( 'NONE', #23904, #108 ) ;
#24036=FACE_OUTER_BOUND ( 'NONE', #11307, .T. ) ;
#24040=CARTESIAN_POINT ( 'NONE',  ( 44.81606138205700063, -34.55876147765400930, 73.30501292737011454 ) ) ;
#24044=ORIENTED_EDGE ( 'NONE', *, *, #20472, .T. ) ;
#24060=EDGE_CURVE ( 'NONE', #17954, #14226, #20184, .T. ) ;
#24065=CARTESIAN_POINT ( 'NONE',  ( 35.31606138205687273, 33.19123852234595518, 61.30501292736990848 ) ) ;
#24068=DIRECTION ( 'NONE',  ( -1.000000000000000000, 0.000000000000000000, 0.000000000000000000 ) ) ;
#24081=PLANE ( 'NONE',  #25064 ) ;
#24094=CARTESIAN_POINT ( 'NONE',  ( 44.81606138205700063, -34.55876147765400930, 73.30501292737011454 ) ) ;
#24101=CARTESIAN_POINT ( 'NONE',  ( 43.81606138205700063, -34.55876147765403061, 66.30501292737011454 ) ) ;
#24104=ORIENTED_EDGE ( 'NONE', *, *, #23926, .F. ) ;
#24110=DIRECTION ( 'NONE',  ( 0.000000000000000000, -1.000000000000000000, 2.999999999999999839E-15 ) ) ;
#24119=DIRECTION ( 'NONE',  ( 0.000000000000000000, 1.000000000000000000, 0.000000000000000000 ) ) ;
#24120=CARTESIAN_POINT ( 'NONE',  ( 44.81606138205700063, -24.55876147765401996, 67.80501292737008612 ) ) ;
#24122=LINE ( 'NONE', #431, #14793 ) ;
#24127=DIRECTION ( 'NONE',  ( -1.000000000000000000, 0.000000000000000000, 0.000000000000000000 ) ) ;
#24128=DIRECTION ( 'NONE',  ( 0.000000000000000000, -1.000000000000000000, 2.999999999999999839E-15 ) ) ;
#24151=CARTESIAN_POINT ( 'NONE',  ( 44.81606138205700063, 41.44123852234595518, 61.30501292736988006 ) ) ;
#24154=DIRECTION ( 'NONE',  ( 1.734723475976805122E-15, 2.999999999999999839E-15, 1.000000000000000000 ) ) ;
#24158=ORIENTED_EDGE ( 'NONE', *, *, #24011, .F. ) ;
#24172=VECTOR ( 'NONE', #6781, 1000.000000000000000 ) ;
#24175=LINE ( 'NONE', #2419, #20245 ) ;
#24176=EDGE_CURVE ( 'NONE', #10990, #5522, #19770, .T. ) ;
#24183=EDGE_LOOP ( 'NONE', ( #4507, #6440, #14610, #9492 ) ) ;
#24196=ORIENTED_EDGE ( 'NONE', *, *, #21284, .T. ) ;
#24197=DIRECTION ( 'NONE',  ( 1.000000000000000000, -5.510910596163088391E-31, -1.836970198721029688E-16 ) ) ;
#24202=DIRECTION ( 'NONE',  ( 0.000000000000000000, 1.000000000000000000, 0.000000000000000000 ) ) ;
#24203=EDGE_CURVE ( 'NONE', #1142, #8061, #17507, .T. ) ;
#24214=VECTOR ( 'NONE', #22898, 1000.000000000000000 ) ;
#24221=DIRECTION ( 'NONE',  ( 0.000000000000000000, -1.000000000000000000, 3.129456975819164530E-15 ) ) ;
#24234=DIRECTION ( 'NONE',  ( 0.000000000000000000, 1.000000000000000000, -5.551115123125785858E-15 ) ) ;
#24244=CIRCLE ( 'NONE', #5353, 0.7500000000000006661 ) ;
#24257=CARTESIAN_POINT ( 'NONE',  ( 31.81606138205700418, 18.19123852234599070, 72.05501292736995822 ) ) ;
#24261=ORIENTED_EDGE ( 'NONE', *, *, #16102, .T. ) ;
#24264=DIRECTION ( 'NONE',  ( -1.000000000000000000, 1.040834085586084551E-30, 3.469446951953615175E-16 ) ) ;
#24272=EDGE_CURVE ( 'NONE', #15369, #14131, #18142, .T. ) ;
#24273=LINE ( 'NONE', #4210, #7280 ) ;
#24274=EDGE_LOOP ( 'NONE', ( #14504, #24104, #25047, #11938 ) ) ;
#24275=EDGE_LOOP ( 'NONE', ( #8537, #10913, #20727, #22350 ) ) ;
#24280=CARTESIAN_POINT ( 'NONE',  ( 40.31606138205700773, 41.44123852234599781, 75.30501292736987295 ) ) ;
#24282=VECTOR ( 'NONE', #22655, 1000.000000000000000 ) ;
#24296=DIRECTION ( 'NONE',  ( 1.000000000000000000, 0.000000000000000000, 0.000000000000000000 ) ) ;
#24299=LINE ( 'NONE', #16712, #12057 ) ;
#24301=DIRECTION ( 'NONE',  ( 1.000000000000000000, 0.000000000000000000, 0.000000000000000000 ) ) ;
#24311=DIRECTION ( 'NONE',  ( 3.306316923293080268E-47, 1.000000000000000000, -2.999999999999999839E-15 ) ) ;
#24313=VERTEX_POINT ( 'NONE', #12349 ) ;
#24321=DIRECTION ( 'NONE',  ( -1.000000000000000000, 1.115179377413661005E-30, 3.717264591378870232E-16 ) ) ;
#24326=EDGE_CURVE ( 'NONE', #1244, #20311, #2524, .T. ) ;
#24328=CYLINDRICAL_SURFACE ( 'NONE', #9166, 2.000000000000001776 ) ;
#24333=CARTESIAN_POINT ( 'NONE',  ( 32.81606138205700773, -34.55876147765400219, 75.30501292737011454 ) ) ;
#24349=CARTESIAN_POINT ( 'NONE',  ( 31.81606138205700418, 39.19123852234599070, 72.05501292736988717 ) ) ;
#24359=EDGE_CURVE ( 'NONE', #2525, #2891, #19939, .T. ) ;
#24363=DIRECTION ( 'NONE',  ( 0.000000000000000000, 1.000000000000000000, -2.999999999999999839E-15 ) ) ;
#24378=ORIENTED_EDGE ( 'NONE', *, *, #11929, .F. ) ;
#24381=VECTOR ( 'NONE', #13446, 1000.000000000000000 ) ;
#24384=ORIENTED_EDGE ( 'NONE', *, *, #8300, .F. ) ;
#24385=DIRECTION ( 'NONE',  ( -1.000000000000000000, 1.301042606982604506E-30, 4.336808689942015271E-16 ) ) ;
#24391=ORIENTED_EDGE ( 'NONE', *, *, #20749, .F. ) ;
#24394=LINE ( 'NONE', #2749, #12051 ) ;
#24402=DIRECTION ( 'NONE',  ( 0.000000000000000000, 1.000000000000000000, 0.000000000000000000 ) ) ;
#24406=CARTESIAN_POINT ( 'NONE',  ( 31.81606138205700418, 41.44123852234599070, 73.55501292736987295 ) ) ;
#24408=DIRECTION ( 'NONE',  ( 1.000000000000000000, 0.000000000000000000, 0.000000000000000000 ) ) ;
#24409=DIRECTION ( 'NONE',  ( 1.000000000000000000, 0.000000000000000000, 0.000000000000000000 ) ) ;
#24412=DIRECTION ( 'NONE',  ( 0.000000000000000000, 1.000000000000000000, 0.000000000000000000 ) ) ;
#24423=EDGE_LOOP ( 'NONE', ( #21700, #1214, #16088, #17468 ) ) ;
#24424=ORIENTED_EDGE ( 'NONE', *, *, #20472, .F. ) ;
#24433=LINE ( 'NONE', #10930, #10833 ) ;
#24451=CARTESIAN_POINT ( 'NONE',  ( 44.81606138205700063, 38.19123852234599070, 73.05501292736988717 ) ) ;
#24462=CARTESIAN_POINT ( 'NONE',  ( 40.31606138205700773, -29.30876147765400574, 73.55501292737010033 ) ) ;
#24465=CARTESIAN_POINT ( 'NONE',  ( 34.81606138205687273, 43.19123852234595518, 61.80501292736988006 ) ) ;
#24475=ORIENTED_EDGE ( 'NONE', *, *, #6900, .F. ) ;
#24485=VERTEX_POINT ( 'NONE', #4851 ) ;
#24486=CARTESIAN_POINT ( 'NONE',  ( 43.81606138205700063, 38.19123852234599070, 72.05501292736988717 ) ) ;
#24490=DIRECTION ( 'NONE',  ( 0.000000000000000000, 0.000000000000000000, 1.000000000000000000 ) ) ;
#24495=ADVANCED_FACE ( 'NONE', ( #1236 ), #16700, .F. ) ;
#24497=EDGE_CURVE ( 'NONE', #9366, #13361, #9514, .T. ) ;
#24501=ORIENTED_EDGE ( 'NONE', *, *, #2927, .F. ) ;
#24503=EDGE_LOOP ( 'NONE', ( #9408, #3642, #20466, #25239 ) ) ;
#24504=EDGE_LOOP ( 'NONE', ( #8738, #18752, #19443, #16377 ) ) ;
#24514=ADVANCED_FACE ( 'NONE', ( #24793, #1362 ), #18510, .T. ) ;
#24524=ADVANCED_FACE ( 'NONE', ( #12604 ), #7559, .T. ) ;
#24538=AXIS2_PLACEMENT_3D ( 'NONE', #10591, #14572, #2707 ) ;
#24542=PLANE ( 'NONE',  #19046 ) ;
#24556=LINE ( 'NONE', #2802, #14373 ) ;
#24559=DIRECTION ( 'NONE',  ( -6.223655385022149827E-47, 1.000000000000000000, -2.999999999999999839E-15 ) ) ;
#24567=CIRCLE ( 'NONE', #4020, 2.499999999999998668 ) ;
#24571=DIRECTION ( 'NONE',  ( -0.000000000000000000, -1.000000000000000000, 2.848211695852029218E-15 ) ) ;
#24607=AXIS2_PLACEMENT_3D ( 'NONE', #11264, #18852, #24879 ) ;
#24610=FACE_OUTER_BOUND ( 'NONE', #19135, .T. ) ;
#24612=ORIENTED_EDGE ( 'NONE', *, *, #10533, .T. ) ;
#24617=DIRECTION ( 'NONE',  ( -1.000000000000000000, 5.510910596163088391E-31, 1.836970198721029688E-16 ) ) ;
#24618=AXIS2_PLACEMENT_3D ( 'NONE', #20982, #16460, #8884 ) ;
#24620=CARTESIAN_POINT ( 'NONE',  ( 35.81606138205700063, 37.44123852234599781, 75.30501292736990138 ) ) ;
#24625=CIRCLE ( 'NONE', #1195, 0.5000000000000004441 ) ;
#24629=LINE ( 'NONE', #3264, #21381 ) ;
#24635=ORIENTED_EDGE ( 'NONE', *, *, #5065, .T. ) ;
#24639=CARTESIAN_POINT ( 'NONE',  ( 36.31606138205700063, 38.69123852234597649, 69.30501292736988717 ) ) ;
#24649=ADVANCED_FACE ( 'NONE', ( #19147 ), #9746, .T. ) ;
#24651=EDGE_LOOP ( 'NONE', ( #24475, #13954, #11190, #20039 ) ) ;
#24656=DIRECTION ( 'NONE',  ( 0.000000000000000000, 4.914813388431354887E-16, -1.000000000000000000 ) ) ;
#24662=CARTESIAN_POINT ( 'NONE',  ( 44.81606138205700063, 35.44123852234597649, 68.80501292736990138 ) ) ;
#24663=AXIS2_PLACEMENT_3D ( 'NONE', #7871, #5668, #11869 ) ;
#24664=CARTESIAN_POINT ( 'NONE',  ( 43.81606138205700063, 41.44123852234599070, 73.30501292736985874 ) ) ;
#24668=DIRECTION ( 'NONE',  ( 1.000000000000000000, 0.000000000000000000, 0.000000000000000000 ) ) ;
#24682=VECTOR ( 'NONE', #14796, 1000.000000000000000 ) ;
#24688=FACE_OUTER_BOUND ( 'NONE', #23892, .T. ) ;
#24696=LINE ( 'NONE', #9013, #24682 ) ;
#24697=ORIENTED_EDGE ( 'NONE', *, *, #12959, .T. ) ;
#24711=DIRECTION ( 'NONE',  ( 0.000000000000000000, 0.000000000000000000, 1.000000000000000000 ) ) ;
#24726=CARTESIAN_POINT ( 'NONE',  ( 38.31606138205700063, 42.51966564709218233, 70.30501292737018559 ) ) ;
#24731=VERTEX_POINT ( 'NONE', #15904 ) ;
#24743=FACE_BOUND ( 'NONE', #21563, .T. ) ;
#24752=AXIS2_PLACEMENT_3D ( 'NONE', #6038, #95, #13771 ) ;
#24772=AXIS2_PLACEMENT_3D ( 'NONE', #21759, #1183, #16917 ) ;
#24778=ORIENTED_EDGE ( 'NONE', *, *, #24359, .T. ) ;
#24779=CARTESIAN_POINT ( 'NONE',  ( 31.81606138205700418, -34.55876147765403061, 66.30501292737011454 ) ) ;
#24782=DIRECTION ( 'NONE',  ( 1.000000000000000000, 0.000000000000000000, 0.000000000000000000 ) ) ;
#24785=ORIENTED_EDGE ( 'NONE', *, *, #2194, .T. ) ;
#24793=FACE_BOUND ( 'NONE', #18779, .T. ) ;
#24796=LINE ( 'NONE', #23005, #12855 ) ;
#24801=AXIS2_PLACEMENT_3D ( 'NONE', #456, #8083, #10017 ) ;
#24817=DIRECTION ( 'NONE',  ( 0.000000000000000000, 2.848211695852029218E-15, 1.000000000000000000 ) ) ;
#24818=FACE_BOUND ( 'NONE', #16138, .T. ) ;
#24825=DIRECTION ( 'NONE',  ( -1.000000000000000000, 0.000000000000000000, 0.000000000000000000 ) ) ;
#24831=EDGE_CURVE ( 'NONE', #20324, #8796, #11937, .T. ) ;
#24835=ORIENTED_EDGE ( 'NONE', *, *, #12811, .T. ) ;
#24838=EDGE_CURVE ( 'NONE', #17124, #13011, #8315, .T. ) ;
#24846=CARTESIAN_POINT ( 'NONE',  ( 44.81606138205700063, -33.00876147765401925, 70.30501292737011454 ) ) ;
#24849=AXIS2_PLACEMENT_3D ( 'NONE', #285, #12555, #6365 ) ;
#24871=CARTESIAN_POINT ( 'NONE',  ( 32.81606138205700773, -36.55876147765400930, 73.30501292737011454 ) ) ;
#24872=DIRECTION ( 'NONE',  ( -1.000000000000000000, 1.115179377413661005E-30, 3.717264591378870232E-16 ) ) ;
#24879=DIRECTION ( 'NONE',  ( 0.000000000000000000, 1.000000000000000000, 0.000000000000000000 ) ) ;
#24883=ORIENTED_EDGE ( 'NONE', *, *, #10200, .F. ) ;
#24891=CARTESIAN_POINT ( 'NONE',  ( 32.81606138205700773, 41.44123852234599070, 73.55501292736987295 ) ) ;
#24902=LINE ( 'NONE', #21195, #7155 ) ;
#24904=CARTESIAN_POINT ( 'NONE',  ( 43.06606138205700063, 42.19123852234601202, 79.18605660143489899 ) ) ;
#24910=ORIENTED_EDGE ( 'NONE', *, *, #7509, .F. ) ;
#24914=ORIENTED_EDGE ( 'NONE', *, *, #7661, .F. ) ;
#24917=DIRECTION ( 'NONE',  ( 0.000000000000000000, -1.000000000000000000, 0.000000000000000000 ) ) ;
#24927=VERTEX_POINT ( 'NONE', #7689 ) ;
#24930=CARTESIAN_POINT ( 'NONE',  ( 33.56606138205700773, 41.44123852234599781, 75.30501292736988717 ) ) ;
#24933=CARTESIAN_POINT ( 'NONE',  ( 35.81606138205700063, 41.44123852234599781, 75.30501292736988717 ) ) ;
#24935=FACE_OUTER_BOUND ( 'NONE', #14999, .T. ) ;
#24937=VECTOR ( 'NONE', #4290, 1000.000000000000000 ) ;
#24939=CARTESIAN_POINT ( 'NONE',  ( 40.31606138205700773, 39.69123852234597649, 69.30501292736988717 ) ) ;
#24940=EDGE_CURVE ( 'NONE', #3119, #5370, #11566, .T. ) ;
#24957=AXIS2_PLACEMENT_3D ( 'NONE', #6337, #19988, #21917 ) ;
#24964=ADVANCED_FACE ( 'NONE', ( #5624 ), #1740, .T. ) ;
#24965=CARTESIAN_POINT ( 'NONE',  ( 43.06606138205700063, 42.19123852234599070, 73.55501292736987295 ) ) ;
#24971=EDGE_CURVE ( 'NONE', #19274, #18444, #9260, .T. ) ;
#24985=EDGE_CURVE ( 'NONE', #6436, #21126, #21467, .T. ) ;
#24988=CARTESIAN_POINT ( 'NONE',  ( 44.81606138205700063, 41.44123852234599781, 75.30501292736987295 ) ) ;
#25002=CARTESIAN_POINT ( 'NONE',  ( 32.81606138205700773, -34.55876147765400930, 73.30501292737011454 ) ) ;
#25005=CARTESIAN_POINT ( 'NONE',  ( 43.81606138205700063, 28.69846577177642288, 66.12638289304319983 ) ) ;
#25016=ORIENTED_EDGE ( 'NONE', *, *, #16919, .F. ) ;
#25023=DIRECTION ( 'NONE',  ( 0.000000000000000000, -1.000000000000000000, 2.999999999999999839E-15 ) ) ;
#25047=ORIENTED_EDGE ( 'NONE', *, *, #24326, .F. ) ;
#25050=FACE_OUTER_BOUND ( 'NONE', #11973, .T. ) ;
#25062=PLANE ( 'NONE',  #16411 ) ;
#25064=AXIS2_PLACEMENT_3D ( 'NONE', #4523, #14435, #16103 ) ;
#25065=LINE ( 'NONE', #7449, #1210 ) ;
#25067=DIRECTION ( 'NONE',  ( 0.000000000000000000, 2.999999999999999839E-15, 1.000000000000000000 ) ) ;
#25085=DIRECTION ( 'NONE',  ( 1.000000000000000000, 2.104045878896135585E-30, -1.734723475976805122E-15 ) ) ;
#25086=EDGE_CURVE ( 'NONE', #8442, #17440, #7953, .T. ) ;
#25089=CARTESIAN_POINT ( 'NONE',  ( 33.56606138205700773, 42.19123852234595518, 61.30501292736988006 ) ) ;
#25099=EDGE_CURVE ( 'NONE', #1199, #22825, #11820, .T. ) ;
#25103=ORIENTED_EDGE ( 'NONE', *, *, #4361, .T. ) ;
#25110=CARTESIAN_POINT ( 'NONE',  ( 44.81606138205700063, -24.55876147765400574, 72.80501292737008612 ) ) ;
#25114=CARTESIAN_POINT ( 'NONE',  ( 43.81606138205700063, 18.19123852234598715, 71.05501292736995822 ) ) ;
#25133=ORIENTED_EDGE ( 'NONE', *, *, #6905, .T. ) ;
#25140=ADVANCED_FACE ( 'NONE', ( #8326 ), #21974, .F. ) ;
#25142=ORIENTED_EDGE ( 'NONE', *, *, #21227, .T. ) ;
#25149=LINE ( 'NONE', #7663, #8554 ) ;
#25151=VERTEX_POINT ( 'NONE', #2383 ) ;
#25152=VERTEX_POINT ( 'NONE', #10257 ) ;
#25167=EDGE_LOOP ( 'NONE', ( #8731, #4667 ) ) ;
#25168=AXIS2_PLACEMENT_3D ( 'NONE', #14911, #5518, #17623 ) ;
#25173=EDGE_LOOP ( 'NONE', ( #9376, #10812, #18236, #16795 ) ) ;
#25186=CARTESIAN_POINT ( 'NONE',  ( 40.31606138205700773, 38.69123852234597649, 69.30501292736988717 ) ) ;
#25199=DIRECTION ( 'NONE',  ( 0.000000000000000000, -1.000000000000000000, 2.999999999999999839E-15 ) ) ;
#25210=ORIENTED_EDGE ( 'NONE', *, *, #9293, .F. ) ;
#25215=ORIENTED_EDGE ( 'NONE', *, *, #21979, .F. ) ;
#25216=DIRECTION ( 'NONE',  ( 0.000000000000000000, 1.163336342344340343E-15, -1.000000000000000000 ) ) ;
#25233=EDGE_LOOP ( 'NONE', ( #2705, #4162, #17442, #1712, #11336 ) ) ;
#25239=ORIENTED_EDGE ( 'NONE', *, *, #23401, .T. ) ;
#25240=DIRECTION ( 'NONE',  ( 1.000000000000000000, 3.083952846180988900E-15, -3.854941057726327830E-16 ) ) ;
#25243=CARTESIAN_POINT ( 'NONE',  ( 44.81606138205700063, 1.441238522345979600, 68.80501292737000085 ) ) ;
#25245=DIRECTION ( 'NONE',  ( 1.000000000000000000, 0.000000000000000000, 0.000000000000000000 ) ) ;
#25246=CARTESIAN_POINT ( 'NONE',  ( 36.31606138205700063, 37.44123852234599781, 75.30501292736988717 ) ) ;
#25254=VERTEX_POINT ( 'NONE', #24639 ) ;
#25262=VECTOR ( 'NONE', #22826, 1000.000000000000000 ) ;
#25272=CARTESIAN_POINT ( 'NONE',  ( 38.31606138205700063, -30.30876147765401285, 71.30501292737010033 ) ) ;
#25276=DIRECTION ( 'NONE',  ( 0.000000000000000000, 1.000000000000000000, 0.000000000000000000 ) ) ;
#25278=ORIENTED_EDGE ( 'NONE', *, *, #1528, .T. ) ;
#25282=DIRECTION ( 'NONE',  ( 0.000000000000000000, 1.000000000000000000, -2.999999999999999839E-15 ) ) ;
#25304=VERTEX_POINT ( 'NONE', #7658 ) ;
#25312=LINE ( 'NONE', #13743, #3722 ) ;
#25324=CARTESIAN_POINT ( 'NONE',  ( 43.81606138205700063, 38.19123852234598360, 71.05501292736988717 ) ) ;
#25330=DIRECTION ( 'NONE',  ( 0.000000000000000000, -1.000000000000000000, 0.000000000000000000 ) ) ;
#25332=EDGE_LOOP ( 'NONE', ( #4760, #18734, #23225, #3326 ) ) ;
#25335=FACE_OUTER_BOUND ( 'NONE', #216, .T. ) ;
#25340=EDGE_CURVE ( 'NONE', #21491, #21773, #17194, .T. ) ;
#25341=CARTESIAN_POINT ( 'NONE',  ( 43.81606138205700063, 41.44123852234595518, 61.30501292736988006 ) ) ;
#25346=CARTESIAN_POINT ( 'NONE',  ( 43.81606138205700063, -34.55876147765401640, 70.30501292737011454 ) ) ;
#25358=VERTEX_POINT ( 'NONE', #5467 ) ;
#25363=CARTESIAN_POINT ( 'NONE',  ( 44.81606138205700063, 41.44123852234599781, 74.30501292736987295 ) ) ;
#25371=DIRECTION ( 'NONE',  ( 0.000000000000000000, 1.000000000000000000, 0.000000000000000000 ) ) ;
#25381=AXIS2_PLACEMENT_3D ( 'NONE', #18963, #12793, #9188 ) ;
#25395=LINE ( 'NONE', #21426, #5894 ) ;
#25399=DIRECTION ( 'NONE',  ( 0.000000000000000000, 1.000000000000000000, 0.000000000000000000 ) ) ;
#25409=EDGE_LOOP ( 'NONE', ( #90, #17901, #24158, #10542 ) ) ;
#25415=CARTESIAN_POINT ( 'NONE',  ( 36.31606138205700063, 38.69123852234599070, 73.55501292736988717 ) ) ;
#25426=DIRECTION ( 'NONE',  ( 0.000000000000000000, -2.913263826201159484E-15, -1.000000000000000000 ) ) ;
#25437=EDGE_LOOP ( 'NONE', ( #7680, #10510, #2462, #18497 ) ) ;
#25449=VECTOR ( 'NONE', #22205, 1000.000000000000000 ) ;
#25474=DIRECTION ( 'NONE',  ( 0.000000000000000000, -1.000000000000000000, 2.999999999999999839E-15 ) ) ;
#25477=VECTOR ( 'NONE', #4977, 1000.000000000000000 ) ;
#25478=( LENGTH_UNIT ( ) NAMED_UNIT ( * ) SI_UNIT ( .MILLI., .METRE. ) );
#25479=CARTESIAN_POINT ( 'NONE',  ( 35.81606138205700063, 37.44123852234599781, 74.30501292736988717 ) ) ;
#25480=EDGE_CURVE ( 'NONE', #4935, #17850, #11788, .T. ) ;
ENDSEC;
END-ISO-10303-21;
